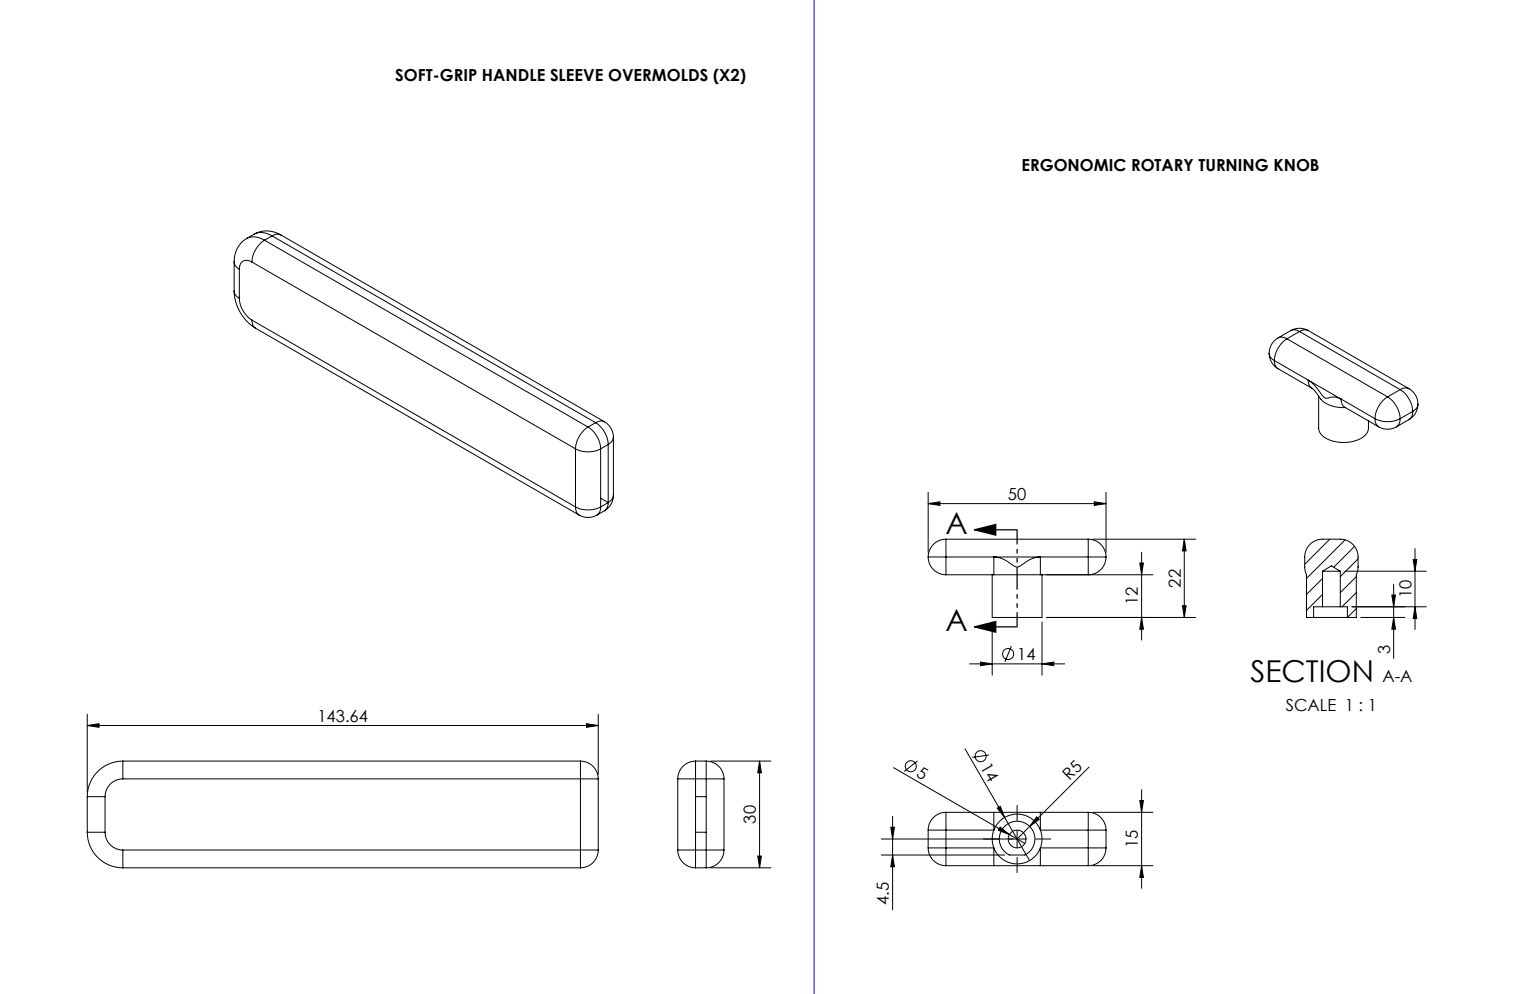
ISO-10303-21;
HEADER;
FILE_DESCRIPTION (('STEP AP214'),
    '1' );
FILE_NAME ('Soft-Grip Handle Sleeve Overmolds (x2).step',
    '2026-09-24T10:15:42',
    ( '' ),
    ( '' ),
    'SwSTEP 2.0',
    'SolidWorks 2026',
    '' );
FILE_SCHEMA (( 'AUTOMOTIVE_DESIGN' ));
ENDSEC;

DATA;
#10=DIRECTION ( 'NONE',  ( -0.000000000000000000, 1.000000000000000000, -0.000000000000000000 ) ) ;
#45=( NAMED_UNIT ( * ) PLANE_ANGLE_UNIT ( ) SI_UNIT ( $, .RADIAN. ) );
#53=DIRECTION ( 'NONE',  ( 0.000000000000000000, 0.000000000000000000, 1.000000000000000000 ) ) ;
#71=EDGE_CURVE ( 'NONE', #14216, #17792, #8218, .T. ) ;
#74=EDGE_CURVE ( 'NONE', #18124, #2507, #14609, .T. ) ;
#81=ORIENTED_EDGE ( 'NONE', *, *, #18589, .F. ) ;
#107=AXIS2_PLACEMENT_3D ( 'NONE', #8749, #9037, #10469 ) ;
#121=FACE_OUTER_BOUND ( 'NONE', #17396, .T. ) ;
#125=ORIENTED_EDGE ( 'NONE', *, *, #5943, .T. ) ;
#129=EDGE_CURVE ( 'NONE', #11279, #879, #18664, .T. ) ;
#146=( NAMED_UNIT ( * ) PLANE_ANGLE_UNIT ( ) SI_UNIT ( $, .RADIAN. ) );
#165=ORIENTED_EDGE ( 'NONE', *, *, #2738, .T. ) ;
#168=DIRECTION ( 'NONE',  ( 2.775557561562891351E-15, 0.000000000000000000, -1.000000000000000000 ) ) ;
#195=EDGE_CURVE ( 'NONE', #996, #10455, #10657, .T. ) ;
#204=VERTEX_POINT ( 'NONE', #4724 ) ;
#216=AXIS2_PLACEMENT_3D ( 'NONE', #4197, #14959, #10013 ) ;
#297=ADVANCED_FACE ( 'NONE', ( #11306 ), #18192, .T. ) ;
#339=( NAMED_UNIT ( * ) SI_UNIT ( $, .STERADIAN. ) SOLID_ANGLE_UNIT ( ) );
#364=CARTESIAN_POINT ( 'NONE',  ( -199.9999999999999716, -10.00000000000002665, 6.000000000000000000 ) ) ;
#368=PRODUCT_DEFINITION_SHAPE ( 'NONE', 'NONE',  #14430 ) ;
#400=VERTEX_POINT ( 'NONE', #4028 ) ;
#441=VECTOR ( 'NONE', #16423, 1000.000000000000000 ) ;
#456=ORIENTED_EDGE ( 'NONE', *, *, #3384, .T. ) ;
#478=DIRECTION ( 'NONE',  ( -1.000000000000000000, -1.298018465182616140E-16, -0.000000000000000000 ) ) ;
#495=ORIENTED_EDGE ( 'NONE', *, *, #13811, .F. ) ;
#571=ORIENTED_EDGE ( 'NONE', *, *, #13222, .F. ) ;
#632=DIRECTION ( 'NONE',  ( 0.000000000000000000, 0.000000000000000000, -1.000000000000000000 ) ) ;
#645=EDGE_CURVE ( 'NONE', #12951, #4745, #12694, .T. ) ;
#673=DIRECTION ( 'NONE',  ( 1.000000000000000000, 0.000000000000000000, -0.000000000000000000 ) ) ;
#681=AXIS2_PLACEMENT_3D ( 'NONE', #16263, #10, #9092 ) ;
#709=CYLINDRICAL_SURFACE ( 'NONE', #9338, 5.000000000000000000 ) ;
#710=CARTESIAN_POINT ( 'NONE',  ( -199.9999999999999716, -5.000000000000024869, 3.000000000000000000 ) ) ;
#723=EDGE_CURVE ( 'NONE', #14183, #11279, #13412, .T. ) ;
#729=EDGE_LOOP ( 'NONE', ( #5711, #14745, #14272, #12333 ) ) ;
#732=FACE_OUTER_BOUND ( 'NONE', #9253, .T. ) ;
#733=CARTESIAN_POINT ( 'NONE',  ( -66.35602477868049220, -15.00000000000001066, -153.7432847437423789 ) ) ;
#741=LINE ( 'NONE', #9527, #14448 ) ;
#746=ORIENTED_EDGE ( 'NONE', *, *, #8212, .T. ) ;
#763=LINE ( 'NONE', #18253, #3069 ) ;
#778=ORIENTED_EDGE ( 'NONE', *, *, #1912, .F. ) ;
#783=CARTESIAN_POINT ( 'NONE',  ( -194.9999999999999716, 4.999999999999973355, 6.000000000000000000 ) ) ;
#830=COLOUR_RGB ( '', 0.08235294, 0.09019608, 0.10196078) ;
#879=VERTEX_POINT ( 'NONE', #5706 ) ;
#880=DIRECTION ( 'NONE',  ( 1.000000000000000000, 1.298018465182616140E-16, 0.000000000000000000 ) ) ;
#921=LINE ( 'NONE', #8015, #14130 ) ;
#932=DIRECTION ( 'NONE',  ( -1.000000000000000000, 0.000000000000000000, 0.000000000000000000 ) ) ;
#947=ORIENTED_EDGE ( 'NONE', *, *, #11281, .T. ) ;
#949=EDGE_CURVE ( 'NONE', #14986, #8583, #5172, .T. ) ;
#979=LINE ( 'NONE', #3397, #6527 ) ;
#996=VERTEX_POINT ( 'NONE', #10503 ) ;
#1017=CARTESIAN_POINT ( 'NONE',  ( -194.9999999999999716, 4.999999999999973355, 11.00000000000000000 ) ) ;
#1053=CARTESIAN_POINT ( 'NONE',  ( -194.9999999999999716, -15.00000000000003020, -153.7432847437423789 ) ) ;
#1169=CARTESIAN_POINT ( 'NONE',  ( -194.9999999999999716, -10.00000000000002665, 11.00000000000000000 ) ) ;
#1263=CARTESIAN_POINT ( 'NONE',  ( -194.9999999999999716, 9.999999999999973355, 3.000000000000000000 ) ) ;
#1267=DIRECTION ( 'NONE',  ( -0.000000000000000000, -0.000000000000000000, 1.000000000000000000 ) ) ;
#1290=AXIS2_PLACEMENT_3D ( 'NONE', #1861, #1565, #7701 ) ;
#1301=CARTESIAN_POINT ( 'NONE',  ( -61.35602477868049220, 9.999999999999973355, 6.000000000000000000 ) ) ;
#1311=CARTESIAN_POINT ( 'NONE',  ( -61.35602477868047799, -10.00000000000000888, -153.7432847437423789 ) ) ;
#1312=EDGE_CURVE ( 'NONE', #1583, #8583, #4177, .T. ) ;
#1314=ORIENTED_EDGE ( 'NONE', *, *, #723, .T. ) ;
#1317=CYLINDRICAL_SURFACE ( 'NONE', #216, 5.000000000000000000 ) ;
#1334=CARTESIAN_POINT ( 'NONE',  ( 1.298018465182615993E-15, -10.00000000000000000, -2.000000000000000000 ) ) ;
#1355=CARTESIAN_POINT ( 'NONE',  ( 0.000000000000000000, 0.000000000000000000, 6.000000000000000000 ) ) ;
#1371=AXIS2_PLACEMENT_3D ( 'NONE', #17480, #5906, #4386 ) ;
#1389=DIRECTION ( 'NONE',  ( -0.000000000000000000, 0.000000000000000000, -1.000000000000000000 ) ) ;
#1393=ORIENTED_EDGE ( 'NONE', *, *, #11938, .T. ) ;
#1436=CARTESIAN_POINT ( 'NONE',  ( -194.9999999999999716, -10.00000000000002665, -2.000000000000000000 ) ) ;
#1460=CIRCLE ( 'NONE', #12158, 5.000000000000000000 ) ;
#1465=CARTESIAN_POINT ( 'NONE',  ( -66.35602477868047799, 9.999999999999973355, -2.000000000000000000 ) ) ;
#1474=EDGE_CURVE ( 'NONE', #11944, #7533, #979, .T. ) ;
#1485=CARTESIAN_POINT ( 'NONE',  ( -194.9999999999999716, 14.99999999999997513, 6.000000000000005329 ) ) ;
#1487=( LENGTH_UNIT ( ) NAMED_UNIT ( * ) SI_UNIT ( .MILLI., .METRE. ) );
#1496=ORIENTED_EDGE ( 'NONE', *, *, #18440, .T. ) ;
#1498=ORIENTED_EDGE ( 'NONE', *, *, #9213, .F. ) ;
#1512=DIRECTION ( 'NONE',  ( 0.000000000000000000, 0.000000000000000000, -1.000000000000000000 ) ) ;
#1558=ORIENTED_EDGE ( 'NONE', *, *, #2425, .T. ) ;
#1563=CARTESIAN_POINT ( 'NONE',  ( -194.9999999999999716, -10.00000000000002665, 6.000000000000000000 ) ) ;
#1565=DIRECTION ( 'NONE',  ( 0.000000000000000000, 0.000000000000000000, -1.000000000000000000 ) ) ;
#1583=VERTEX_POINT ( 'NONE', #11396 ) ;
#1593=CARTESIAN_POINT ( 'NONE',  ( -205.0000000000000000, 4.999999999999975131, 3.000000000000002665 ) ) ;
#1621=DIRECTION ( 'NONE',  ( 1.000000000000000000, 0.000000000000000000, 0.000000000000000000 ) ) ;
#1625=ORIENTED_EDGE ( 'NONE', *, *, #5264, .F. ) ;
#1702=ORIENTED_EDGE ( 'NONE', *, *, #5723, .T. ) ;
#1765=( LENGTH_UNIT ( ) NAMED_UNIT ( * ) SI_UNIT ( .MILLI., .METRE. ) );
#1782=ORIENTED_EDGE ( 'NONE', *, *, #7144, .F. ) ;
#1799=PLANE ( 'NONE',  #7889 ) ;
#1861=CARTESIAN_POINT ( 'NONE',  ( 0.000000000000000000, 0.000000000000000000, 3.000000000000000000 ) ) ;
#1912=EDGE_CURVE ( 'NONE', #15844, #11944, #5028, .T. ) ;
#2027=DIRECTION ( 'NONE',  ( -1.000000000000000000, 0.000000000000000000, 0.000000000000000000 ) ) ;
#2030=AXIS2_PLACEMENT_3D ( 'NONE', #15716, #11248, #17249 ) ;
#2035=DIRECTION ( 'NONE',  ( 1.000000000000000000, -0.000000000000000000, 0.000000000000000000 ) ) ;
#2097=EDGE_LOOP ( 'NONE', ( #13783, #6508, #11629, #2309 ) ) ;
#2114=DIRECTION ( 'NONE',  ( 0.000000000000000000, 0.000000000000000000, -1.000000000000000000 ) ) ;
#2149=CARTESIAN_POINT ( 'NONE',  ( -194.9999999999999716, -10.00000000000002665, 5.999999999999999112 ) ) ;
#2213=CYLINDRICAL_SURFACE ( 'NONE', #13097, 10.00000000000000888 ) ;
#2265=ORIENTED_EDGE ( 'NONE', *, *, #8107, .F. ) ;
#2286=LINE ( 'NONE', #16550, #9676 ) ;
#2293=CARTESIAN_POINT ( 'NONE',  ( -194.9999999999999716, -5.000000000000024869, 6.000000000000000000 ) ) ;
#2296=VERTEX_POINT ( 'NONE', #13247 ) ;
#2308=DIRECTION ( 'NONE',  ( -1.000000000000000000, 0.000000000000000000, 0.000000000000000000 ) ) ;
#2309=ORIENTED_EDGE ( 'NONE', *, *, #74, .F. ) ;
#2318=DIRECTION ( 'NONE',  ( -1.000000000000000000, 0.000000000000000000, 0.000000000000000000 ) ) ;
#2331=DIRECTION ( 'NONE',  ( 0.000000000000000000, 0.000000000000000000, 1.000000000000000000 ) ) ;
#2341=ORIENTED_EDGE ( 'NONE', *, *, #6570, .F. ) ;
#2349=CIRCLE ( 'NONE', #17297, 5.000000000000000000 ) ;
#2359=ORIENTED_EDGE ( 'NONE', *, *, #9146, .T. ) ;
#2365=CARTESIAN_POINT ( 'NONE',  ( -194.9999999999999716, -15.00000000000002665, -153.7432847437423789 ) ) ;
#2368=CARTESIAN_POINT ( 'NONE',  ( -194.9999999999999716, 9.999999999999976907, -2.000000000000000000 ) ) ;
#2401=ORIENTED_EDGE ( 'NONE', *, *, #9051, .T. ) ;
#2410=AXIS2_PLACEMENT_3D ( 'NONE', #3830, #2035, #12340 ) ;
#2417=CYLINDRICAL_SURFACE ( 'NONE', #2513, 4.999999999999997335 ) ;
#2425=EDGE_CURVE ( 'NONE', #4745, #12842, #13817, .T. ) ;
#2460=CIRCLE ( 'NONE', #3389, 5.000000000000004441 ) ;
#2462=ADVANCED_FACE ( 'NONE', ( #11521 ), #3966, .T. ) ;
#2496=UNCERTAINTY_MEASURE_WITH_UNIT (LENGTH_MEASURE( 1.000000000000000082E-05 ), #1765, 'distance_accuracy_value', 'NONE');
#2507=VERTEX_POINT ( 'NONE', #7414 ) ;
#2509=ORIENTED_EDGE ( 'NONE', *, *, #7144, .T. ) ;
#2513=AXIS2_PLACEMENT_3D ( 'NONE', #6741, #8534, #5291 ) ;
#2518=DIRECTION ( 'NONE',  ( 1.000000000000000000, 0.000000000000000000, 2.775557561562889773E-15 ) ) ;
#2538=AXIS2_PLACEMENT_3D ( 'NONE', #7054, #5593, #17264 ) ;
#2551=DIRECTION ( 'NONE',  ( 0.000000000000000000, 0.000000000000000000, -1.000000000000000000 ) ) ;
#2557=DIRECTION ( 'NONE',  ( 0.000000000000000000, 1.000000000000000000, 0.000000000000000000 ) ) ;
#2580=AXIS2_PLACEMENT_3D ( 'NONE', #13797, #8261, #5192 ) ;
#2594=DIRECTION ( 'NONE',  ( 1.000000000000000000, 0.000000000000000000, 0.000000000000000000 ) ) ;
#2641=LINE ( 'NONE', #18606, #10242 ) ;
#2659=ORIENTED_EDGE ( 'NONE', *, *, #17064, .F. ) ;
#2710=DIRECTION ( 'NONE',  ( 1.000000000000000000, 0.000000000000000000, 0.000000000000000000 ) ) ;
#2738=EDGE_CURVE ( 'NONE', #11944, #14183, #18292, .T. ) ;
#2752=CYLINDRICAL_SURFACE ( 'NONE', #18758, 5.000000000000000888 ) ;
#2780=CARTESIAN_POINT ( 'NONE',  ( -66.35602477868047799, -10.00000000000000888, -2.000000000000000000 ) ) ;
#2789=ORIENTED_EDGE ( 'NONE', *, *, #129, .T. ) ;
#2929=VECTOR ( 'NONE', #1389, 1000.000000000000000 ) ;
#2933=DIRECTION ( 'NONE',  ( 1.000000000000000000, -2.775557561562892929E-15, 0.000000000000000000 ) ) ;
#2954=ADVANCED_FACE ( 'NONE', ( #16249 ), #3131, .T. ) ;
#2956=ORIENTED_EDGE ( 'NONE', *, *, #18476, .F. ) ;
#2989=( NAMED_UNIT ( * ) SI_UNIT ( $, .STERADIAN. ) SOLID_ANGLE_UNIT ( ) );
#3005=EDGE_LOOP ( 'NONE', ( #15141, #81, #4937, #1625 ) ) ;
#3041=EDGE_LOOP ( 'NONE', ( #9922, #15624, #14342, #4151 ) ) ;
#3069=VECTOR ( 'NONE', #7854, 1000.000000000000000 ) ;
#3070=DIRECTION ( 'NONE',  ( 0.000000000000000000, 0.000000000000000000, -1.000000000000000000 ) ) ;
#3076=SURFACE_STYLE_USAGE ( .BOTH. , #10364 ) ;
#3084=LINE ( 'NONE', #10175, #6365 ) ;
#3124=SPHERICAL_SURFACE ( 'NONE', #14476, 5.000000000000000000 ) ;
#3131=SPHERICAL_SURFACE ( 'NONE', #5399, 5.000000000000000000 ) ;
#3159=EDGE_CURVE ( 'NONE', #4745, #5087, #16034, .T. ) ;
#3176=( NAMED_UNIT ( * ) SI_UNIT ( $, .STERADIAN. ) SOLID_ANGLE_UNIT ( ) );
#3183=DIRECTION ( 'NONE',  ( -0.000000000000000000, 1.000000000000000000, -0.000000000000000000 ) ) ;
#3198=CARTESIAN_POINT ( 'NONE',  ( -59.99999999999997158, -10.00000000000000888, 3.000000000000000000 ) ) ;
#3214=EDGE_LOOP ( 'NONE', ( #4994, #3976, #1782 ) ) ;
#3219=ORIENTED_EDGE ( 'NONE', *, *, #5723, .F. ) ;
#3234=DIRECTION ( 'NONE',  ( 0.000000000000000000, -1.000000000000000000, -0.000000000000000000 ) ) ;
#3259=MECHANICAL_DESIGN_GEOMETRIC_PRESENTATION_REPRESENTATION('',(#8169),#4186);
#3284=DIRECTION ( 'NONE',  ( -1.000000000000000000, -1.239088197126290570E-16, 0.000000000000000000 ) ) ;
#3306=CARTESIAN_POINT ( 'NONE',  ( -194.9999999999999716, -10.00000000000002665, 3.000000000000000000 ) ) ;
#3326=CIRCLE ( 'NONE', #2410, 5.000000000000000000 ) ;
#3355=CARTESIAN_POINT ( 'NONE',  ( -194.9999999999999716, 14.99999999999997513, -153.7432847437423789 ) ) ;
#3360=DIRECTION ( 'NONE',  ( 0.000000000000000000, 0.000000000000000000, 1.000000000000000000 ) ) ;
#3370=EDGE_LOOP ( 'NONE', ( #13830, #15289, #2956 ) ) ;
#3371=DIRECTION ( 'NONE',  ( 0.000000000000000000, 0.000000000000000000, 1.000000000000000000 ) ) ;
#3384=EDGE_CURVE ( 'NONE', #11365, #1583, #16163, .T. ) ;
#3386=APPLICATION_CONTEXT ( 'automotive_design' ) ;
#3389=AXIS2_PLACEMENT_3D ( 'NONE', #9370, #2114, #13759 ) ;
#3397=CARTESIAN_POINT ( 'NONE',  ( -199.9999999999999716, 4.999999999999973355, 6.000000000000000000 ) ) ;
#3488=VECTOR ( 'NONE', #1267, 1000.000000000000000 ) ;
#3542=VERTEX_POINT ( 'NONE', #710 ) ;
#3584=VECTOR ( 'NONE', #18387, 1000.000000000000000 ) ;
#3655=ORIENTED_EDGE ( 'NONE', *, *, #11968, .F. ) ;
#3672=DIRECTION ( 'NONE',  ( -1.239088197126290570E-16, 1.000000000000000000, 0.000000000000000000 ) ) ;
#3728=ORIENTED_EDGE ( 'NONE', *, *, #1474, .T. ) ;
#3773=AXIS2_PLACEMENT_3D ( 'NONE', #10326, #16152, #1621 ) ;
#3792=ORIENTED_EDGE ( 'NONE', *, *, #74, .T. ) ;
#3798=DIRECTION ( 'NONE',  ( 1.298018465182616140E-16, -1.000000000000000000, 0.000000000000000000 ) ) ;
#3808=CARTESIAN_POINT ( 'NONE',  ( -66.35602477868047799, 9.999999999999973355, 5.999999999999999112 ) ) ;
#3809=CARTESIAN_POINT ( 'NONE',  ( -205.0000000000000000, -5.000000000000024869, 6.000000000000005329 ) ) ;
#3829=VECTOR ( 'NONE', #11704, 1000.000000000000000 ) ;
#3830=CARTESIAN_POINT ( 'NONE',  ( -194.9999999999999716, 9.999999999999976907, 3.000000000000000000 ) ) ;
#3893=VERTEX_POINT ( 'NONE', #5074 ) ;
#3918=DIRECTION ( 'NONE',  ( -0.000000000000000000, -0.000000000000000000, 1.000000000000000000 ) ) ;
#3931=AXIS2_PLACEMENT_3D ( 'NONE', #4340, #14651, #14743 ) ;
#3940=ORIENTED_EDGE ( 'NONE', *, *, #13397, .F. ) ;
#3944=DIRECTION ( 'NONE',  ( 0.000000000000000000, 0.000000000000000000, -1.000000000000000000 ) ) ;
#3953=AXIS2_PLACEMENT_3D ( 'NONE', #5234, #15192, #932 ) ;
#3954=CARTESIAN_POINT ( 'NONE',  ( -199.9999999999999716, -5.000000000000024869, 3.000000000000000000 ) ) ;
#3966=CYLINDRICAL_SURFACE ( 'NONE', #7563, 4.999999999999997335 ) ;
#3976=ORIENTED_EDGE ( 'NONE', *, *, #3159, .T. ) ;
#4008=CARTESIAN_POINT ( 'NONE',  ( -199.9999999999999716, 4.999999999999974243, -2.000000000000000000 ) ) ;
#4028=CARTESIAN_POINT ( 'NONE',  ( -199.9999999999999716, 4.999999999999974243, 11.00000000000000000 ) ) ;
#4047=CARTESIAN_POINT ( 'NONE',  ( -194.9999999999999716, 9.999999999999973355, 6.000000000000000000 ) ) ;
#4062=CARTESIAN_POINT ( 'NONE',  ( -205.0000000000000000, 4.999999999999974243, 3.000000000000002665 ) ) ;
#4086=DIRECTION ( 'NONE',  ( -1.000000000000000000, 0.000000000000000000, 0.000000000000000000 ) ) ;
#4096=EDGE_CURVE ( 'NONE', #8123, #10867, #15534, .T. ) ;
#4114=CARTESIAN_POINT ( 'NONE',  ( -194.9999999999999716, 9.999999999999973355, 3.000000000000002665 ) ) ;
#4151=ORIENTED_EDGE ( 'NONE', *, *, #11967, .T. ) ;
#4156=EDGE_LOOP ( 'NONE', ( #15184, #15990, #2659, #571 ) ) ;
#4157=AXIS2_PLACEMENT_3D ( 'NONE', #1017, #8029, #8208 ) ;
#4177=LINE ( 'NONE', #13436, #12921 ) ;
#4179=DIRECTION ( 'NONE',  ( 1.000000000000000000, 0.000000000000000000, -0.000000000000000000 ) ) ;
#4186=( GEOMETRIC_REPRESENTATION_CONTEXT ( 3 ) GLOBAL_UNCERTAINTY_ASSIGNED_CONTEXT ( ( #2496 ) ) GLOBAL_UNIT_ASSIGNED_CONTEXT ( ( #1765, #6067, #3176 ) ) REPRESENTATION_CONTEXT ( 'NONE', 'WORKASPACE' ) );
#4189=CLOSED_SHELL ( 'NONE', ( #297, #7987, #9459, #11355, #4727, #17066, #8467, #18898, #9820, #4892, #7667, #11879, #11295, #14268, #8812, #8260, #18591, #14598, #18465, #18406, #2462, #16106, #2954, #16000, #18217, #9314, #7143, #4861, #13549, #11149, #9662, #7236 ) ) ;
#4197=CARTESIAN_POINT ( 'NONE',  ( -199.9999999999999716, 4.999999999999975131, 3.000000000000002665 ) ) ;
#4238=EDGE_CURVE ( 'NONE', #14839, #12842, #11714, .T. ) ;
#4260=DIRECTION ( 'NONE',  ( 0.000000000000000000, 0.000000000000000000, 1.000000000000000000 ) ) ;
#4297=CYLINDRICAL_SURFACE ( 'NONE', #1371, 5.000000000000000000 ) ;
#4298=VERTEX_POINT ( 'NONE', #2368 ) ;
#4340=CARTESIAN_POINT ( 'NONE',  ( -194.9999999999999716, 4.999999999999973355, 3.000000000000002665 ) ) ;
#4375=SPHERICAL_SURFACE ( 'NONE', #8750, 5.000000000000000000 ) ;
#4381=VECTOR ( 'NONE', #10253, 1000.000000000000000 ) ;
#4386=DIRECTION ( 'NONE',  ( 0.000000000000000000, 1.000000000000000000, 0.000000000000000000 ) ) ;
#4388=DIRECTION ( 'NONE',  ( 1.000000000000000000, 0.000000000000000000, 0.000000000000000000 ) ) ;
#4423=ORIENTED_EDGE ( 'NONE', *, *, #10269, .T. ) ;
#4432=CARTESIAN_POINT ( 'NONE',  ( -194.9999999999999716, -5.000000000000024869, 6.000000000000000000 ) ) ;
#4443=AXIS2_PLACEMENT_3D ( 'NONE', #11088, #12592, #9464 ) ;
#4458=AXIS2_PLACEMENT_3D ( 'NONE', #7767, #17893, #2027 ) ;
#4487=ORIENTED_EDGE ( 'NONE', *, *, #14077, .T. ) ;
#4501=VECTOR ( 'NONE', #880, 1000.000000000000000 ) ;
#4539=EDGE_CURVE ( 'NONE', #10086, #3893, #6235, .T. ) ;
#4553=ORIENTED_EDGE ( 'NONE', *, *, #9404, .T. ) ;
#4573=FACE_OUTER_BOUND ( 'NONE', #3370, .T. ) ;
#4585=DIRECTION ( 'NONE',  ( 0.000000000000000000, 0.000000000000000000, -1.000000000000000000 ) ) ;
#4614=EDGE_CURVE ( 'NONE', #17792, #996, #7535, .T. ) ;
#4670=EDGE_CURVE ( 'NONE', #18124, #4997, #12934, .T. ) ;
#4671=ORIENTED_EDGE ( 'NONE', *, *, #1912, .T. ) ;
#4682=CIRCLE ( 'NONE', #15046, 5.000000000000000000 ) ;
#4685=DIRECTION ( 'NONE',  ( 0.000000000000000000, 0.000000000000000000, -1.000000000000000000 ) ) ;
#4686=CARTESIAN_POINT ( 'NONE',  ( -194.9999999999999716, -15.00000000000003020, 6.000000000000005329 ) ) ;
#4688=EDGE_CURVE ( 'NONE', #2296, #14986, #4708, .T. ) ;
#4700=ORIENTED_EDGE ( 'NONE', *, *, #12074, .F. ) ;
#4708=CIRCLE ( 'NONE', #15382, 5.000000000000000000 ) ;
#4724=CARTESIAN_POINT ( 'NONE',  ( -66.35602477868049220, -10.00000000000000888, 11.00000000000000000 ) ) ;
#4725=EDGE_LOOP ( 'NONE', ( #2509, #11743, #18683, #495 ) ) ;
#4727=ADVANCED_FACE ( 'NONE', ( #4944 ), #6474, .T. ) ;
#4729=FILL_AREA_STYLE ('',( #17632 ) ) ;
#4745=VERTEX_POINT ( 'NONE', #15658 ) ;
#4747=VERTEX_POINT ( 'NONE', #4008 ) ;
#4749=VECTOR ( 'NONE', #18648, 1000.000000000000000 ) ;
#4762=CARTESIAN_POINT ( 'NONE',  ( -66.35602477868047799, 9.999999999999973355, 5.999999999999999112 ) ) ;
#4763=ORIENTED_EDGE ( 'NONE', *, *, #12688, .T. ) ;
#4777=AXIS2_PLACEMENT_3D ( 'NONE', #6838, #8006, #15436 ) ;
#4812=LINE ( 'NONE', #15468, #10950 ) ;
#4835=LINE ( 'NONE', #1334, #16033 ) ;
#4844=ORIENTED_EDGE ( 'NONE', *, *, #4688, .F. ) ;
#4861=ADVANCED_FACE ( 'NONE', ( #13174 ), #5904, .T. ) ;
#4865=ORIENTED_EDGE ( 'NONE', *, *, #11732, .F. ) ;
#4892=ADVANCED_FACE ( 'NONE', ( #13268 ), #8875, .T. ) ;
#4897=ORIENTED_EDGE ( 'NONE', *, *, #15609, .F. ) ;
#4937=ORIENTED_EDGE ( 'NONE', *, *, #17064, .T. ) ;
#4944=FACE_OUTER_BOUND ( 'NONE', #14107, .T. ) ;
#4970=FACE_OUTER_BOUND ( 'NONE', #2097, .T. ) ;
#4982=EDGE_LOOP ( 'NONE', ( #16888, #8730, #17424, #4423, #3792, #15660 ) ) ;
#4994=ORIENTED_EDGE ( 'NONE', *, *, #645, .T. ) ;
#4997=VERTEX_POINT ( 'NONE', #15605 ) ;
#5028=CIRCLE ( 'NONE', #17535, 5.000000000000004441 ) ;
#5035=CARTESIAN_POINT ( 'NONE',  ( -199.9999999999999716, -10.00000000000002665, 3.000000000000000000 ) ) ;
#5048=FACE_OUTER_BOUND ( 'NONE', #12747, .T. ) ;
#5050=EDGE_CURVE ( 'NONE', #11395, #15844, #11233, .T. ) ;
#5074=CARTESIAN_POINT ( 'NONE',  ( -194.9999999999999716, 9.999999999999973355, 11.00000000000000000 ) ) ;
#5087=VERTEX_POINT ( 'NONE', #2780 ) ;
#5109=PRODUCT_CONTEXT ( 'NONE', #8042, 'mechanical' ) ;
#5172=CIRCLE ( 'NONE', #5770, 5.000000000000000000 ) ;
#5177=CARTESIAN_POINT ( 'NONE',  ( -194.9999999999999716, 14.99999999999997513, 3.000000000000002665 ) ) ;
#5179=CARTESIAN_POINT ( 'NONE',  ( -194.9999999999999716, -15.00000000000002665, 3.000000000000002665 ) ) ;
#5192=DIRECTION ( 'NONE',  ( 0.000000000000000000, 0.000000000000000000, 1.000000000000000000 ) ) ;
#5224=CARTESIAN_POINT ( 'NONE',  ( -199.9999999999999716, 4.999999999999973355, 6.000000000000000000 ) ) ;
#5234=CARTESIAN_POINT ( 'NONE',  ( -66.35602477868047799, 9.999999999999973355, 3.000000000000002665 ) ) ;
#5235=DIRECTION ( 'NONE',  ( 1.000000000000000000, 1.298018465182616140E-16, 0.000000000000000000 ) ) ;
#5264=EDGE_CURVE ( 'NONE', #11365, #14216, #12347, .T. ) ;
#5285=AXIS2_PLACEMENT_3D ( 'NONE', #8439, #2331, #2594 ) ;
#5291=DIRECTION ( 'NONE',  ( 1.000000000000000000, 0.000000000000000000, 0.000000000000000000 ) ) ;
#5297=ORIENTED_EDGE ( 'NONE', *, *, #13444, .F. ) ;
#5307=AXIS2_PLACEMENT_3D ( 'NONE', #3306, #9148, #10388 ) ;
#5334=CARTESIAN_POINT ( 'NONE',  ( -66.35602477868047799, -15.00000000000001066, 3.000000000000002665 ) ) ;
#5358=TOROIDAL_SURFACE ( 'NONE', #12676, 5.000000000000005329, 5.000000000000000000 ) ;
#5384=DIRECTION ( 'NONE',  ( 0.000000000000000000, 1.000000000000000000, 0.000000000000000000 ) ) ;
#5390=CIRCLE ( 'NONE', #7858, 5.000000000000000888 ) ;
#5399=AXIS2_PLACEMENT_3D ( 'NONE', #6409, #7851, #4685 ) ;
#5409=CARTESIAN_POINT ( 'NONE',  ( -61.35602477868047799, -10.00000000000000888, 6.000000000000000000 ) ) ;
#5466=EDGE_LOOP ( 'NONE', ( #2341, #1496, #6560 ) ) ;
#5482=CARTESIAN_POINT ( 'NONE',  ( -66.35602477868047799, 9.999999999999973355, 3.000000000000002665 ) ) ;
#5523=CARTESIAN_POINT ( 'NONE',  ( -66.35602477868049220, 9.999999999999973355, 5.999999999999999112 ) ) ;
#5558=ORIENTED_EDGE ( 'NONE', *, *, #9939, .F. ) ;
#5575=DIRECTION ( 'NONE',  ( 1.000000000000000000, 0.000000000000000000, 0.000000000000000000 ) ) ;
#5580=VECTOR ( 'NONE', #10132, 1000.000000000000000 ) ;
#5593=DIRECTION ( 'NONE',  ( 1.000000000000000000, 0.000000000000000000, 0.000000000000000000 ) ) ;
#5610=EDGE_CURVE ( 'NONE', #1583, #11395, #2286, .T. ) ;
#5643=DIRECTION ( 'NONE',  ( -0.000000000000000000, -1.000000000000000000, -0.000000000000000000 ) ) ;
#5669=CARTESIAN_POINT ( 'NONE',  ( -61.35602477868047799, -15.00000000000001066, 3.000000000000002665 ) ) ;
#5706=CARTESIAN_POINT ( 'NONE',  ( -194.9999999999999716, -10.00000000000002665, 3.000000000000000000 ) ) ;
#5711=ORIENTED_EDGE ( 'NONE', *, *, #14301, .F. ) ;
#5723=EDGE_CURVE ( 'NONE', #10455, #8123, #5390, .T. ) ;
#5742=DIRECTION ( 'NONE',  ( 0.000000000000000000, 1.000000000000000000, 0.000000000000000000 ) ) ;
#5770=AXIS2_PLACEMENT_3D ( 'NONE', #5523, #14329, #18710 ) ;
#5791=SPHERICAL_SURFACE ( 'NONE', #12083, 5.000000000000000000 ) ;
#5865=SURFACE_STYLE_FILL_AREA ( #7616 ) ;
#5904=PLANE ( 'NONE',  #9883 ) ;
#5906=DIRECTION ( 'NONE',  ( 1.000000000000000000, 1.298018465182616140E-16, 0.000000000000000000 ) ) ;
#5929=UNCERTAINTY_MEASURE_WITH_UNIT (LENGTH_MEASURE( 1.000000000000000082E-05 ), #1487, 'distance_accuracy_value', 'NONE');
#5943=EDGE_CURVE ( 'NONE', #10455, #14367, #15247, .T. ) ;
#5968=PRESENTATION_STYLE_ASSIGNMENT (( #16302 ) ) ;
#5983=( GEOMETRIC_REPRESENTATION_CONTEXT ( 3 ) GLOBAL_UNCERTAINTY_ASSIGNED_CONTEXT ( ( #8993 ) ) GLOBAL_UNIT_ASSIGNED_CONTEXT ( ( #16404, #146, #2989 ) ) REPRESENTATION_CONTEXT ( 'NONE', 'WORKASPACE' ) );
#6003=ORIENTED_EDGE ( 'NONE', *, *, #3159, .F. ) ;
#6017=ORIENTED_EDGE ( 'NONE', *, *, #949, .F. ) ;
#6063=DIRECTION ( 'NONE',  ( 0.000000000000000000, 0.000000000000000000, -1.000000000000000000 ) ) ;
#6067=( NAMED_UNIT ( * ) PLANE_ANGLE_UNIT ( ) SI_UNIT ( $, .RADIAN. ) );
#6102=FACE_OUTER_BOUND ( 'NONE', #8541, .T. ) ;
#6161=ORIENTED_EDGE ( 'NONE', *, *, #13811, .T. ) ;
#6191=DIRECTION ( 'NONE',  ( 1.000000000000000000, 0.000000000000000000, 0.000000000000000000 ) ) ;
#6235=CIRCLE ( 'NONE', #2538, 5.000000000000000000 ) ;
#6305=CARTESIAN_POINT ( 'NONE',  ( -199.9999999999999716, 4.999999999999973355, 5.999999999999999112 ) ) ;
#6355=ORIENTED_EDGE ( 'NONE', *, *, #195, .T. ) ;
#6357=ORIENTED_EDGE ( 'NONE', *, *, #13275, .T. ) ;
#6365=VECTOR ( 'NONE', #3183, 1000.000000000000000 ) ;
#6409=CARTESIAN_POINT ( 'NONE',  ( -66.35602477868047799, 9.999999999999973355, 3.000000000000000000 ) ) ;
#6429=DIRECTION ( 'NONE',  ( 1.000000000000000000, 0.000000000000000000, 0.000000000000000000 ) ) ;
#6460=VECTOR ( 'NONE', #14318, 1000.000000000000000 ) ;
#6474=PLANE ( 'NONE',  #17836 ) ;
#6508=ORIENTED_EDGE ( 'NONE', *, *, #13275, .F. ) ;
#6527=VECTOR ( 'NONE', #3944, 1000.000000000000000 ) ;
#6537=ORIENTED_EDGE ( 'NONE', *, *, #7881, .F. ) ;
#6560=ORIENTED_EDGE ( 'NONE', *, *, #4238, .F. ) ;
#6564=CYLINDRICAL_SURFACE ( 'NONE', #4777, 5.000000000000000000 ) ;
#6565=DIRECTION ( 'NONE',  ( -0.000000000000000000, 0.000000000000000000, 1.000000000000000000 ) ) ;
#6567=CARTESIAN_POINT ( 'NONE',  ( -59.99999999999997158, -10.00000000000000888, 6.000000000000000000 ) ) ;
#6569=VECTOR ( 'NONE', #478, 1000.000000000000000 ) ;
#6570=EDGE_CURVE ( 'NONE', #204, #14839, #14091, .T. ) ;
#6573=CARTESIAN_POINT ( 'NONE',  ( -194.9999999999999716, -10.00000000000003020, 11.00000000000000000 ) ) ;
#6576=DIRECTION ( 'NONE',  ( 0.000000000000000000, 0.000000000000000000, 1.000000000000000000 ) ) ;
#6582=AXIS2_PLACEMENT_3D ( 'NONE', #3355, #13300, #13203 ) ;
#6616=DIRECTION ( 'NONE',  ( 0.000000000000000000, 0.000000000000000000, -1.000000000000000000 ) ) ;
#6658=ORIENTED_EDGE ( 'NONE', *, *, #1474, .F. ) ;
#6684=PLANE ( 'NONE',  #13921 ) ;
#6741=CARTESIAN_POINT ( 'NONE',  ( -66.35602477868049220, -10.00000000000000888, -153.7432847437423789 ) ) ;
#6748=CARTESIAN_POINT ( 'NONE',  ( -205.0000000000000000, 4.999999999999975131, 6.000000000000005329 ) ) ;
#6751=ORIENTED_EDGE ( 'NONE', *, *, #6570, .T. ) ;
#6805=ORIENTED_EDGE ( 'NONE', *, *, #13397, .T. ) ;
#6838=CARTESIAN_POINT ( 'NONE',  ( -194.9999999999999716, 9.999999999999973355, 5.999999999999999112 ) ) ;
#6876=VECTOR ( 'NONE', #12112, 1000.000000000000000 ) ;
#6895=DIRECTION ( 'NONE',  ( 0.000000000000000000, 0.000000000000000000, 1.000000000000000000 ) ) ;
#6901=DIRECTION ( 'NONE',  ( -1.000000000000000000, 0.000000000000000000, -0.000000000000000000 ) ) ;
#6945=CARTESIAN_POINT ( 'NONE',  ( -199.9999999999999716, -5.000000000000024869, 6.000000000000000000 ) ) ;
#6947=CARTESIAN_POINT ( 'NONE',  ( -194.9999999999999716, -5.000000000000024869, 6.000000000000005329 ) ) ;
#6975=ORIENTED_EDGE ( 'NONE', *, *, #10269, .F. ) ;
#6989=DIRECTION ( 'NONE',  ( 0.000000000000000000, 0.000000000000000000, 1.000000000000000000 ) ) ;
#7033=DIRECTION ( 'NONE',  ( 2.775557561562891351E-15, 0.000000000000000000, -1.000000000000000000 ) ) ;
#7054=CARTESIAN_POINT ( 'NONE',  ( -194.9999999999999716, 9.999999999999976907, 6.000000000000005329 ) ) ;
#7126=FACE_OUTER_BOUND ( 'NONE', #18557, .T. ) ;
#7143=ADVANCED_FACE ( 'NONE', ( #16189 ), #13414, .F. ) ;
#7144=EDGE_CURVE ( 'NONE', #12951, #5087, #10766, .T. ) ;
#7179=AXIS2_PLACEMENT_3D ( 'NONE', #783, #6616, #18086 ) ;
#7198=DIRECTION ( 'NONE',  ( 0.000000000000000000, 0.000000000000000000, -1.000000000000000000 ) ) ;
#7207=( GEOMETRIC_REPRESENTATION_CONTEXT ( 3 ) GLOBAL_UNCERTAINTY_ASSIGNED_CONTEXT ( ( #5929 ) ) GLOBAL_UNIT_ASSIGNED_CONTEXT ( ( #1487, #45, #339 ) ) REPRESENTATION_CONTEXT ( 'NONE', 'WORKASPACE' ) );
#7215=ORIENTED_EDGE ( 'NONE', *, *, #2738, .F. ) ;
#7221=EDGE_LOOP ( 'NONE', ( #4487, #6537, #18328, #12753 ) ) ;
#7236=ADVANCED_FACE ( 'NONE', ( #11695 ), #17523, .F. ) ;
#7270=DIRECTION ( 'NONE',  ( -0.000000000000000000, -0.000000000000000000, 1.000000000000000000 ) ) ;
#7336=ORIENTED_EDGE ( 'NONE', *, *, #5050, .F. ) ;
#7409=ORIENTED_EDGE ( 'NONE', *, *, #5610, .T. ) ;
#7414=CARTESIAN_POINT ( 'NONE',  ( -199.9999999999999716, -5.000000000000024869, -2.000000000000000000 ) ) ;
#7416=CARTESIAN_POINT ( 'NONE',  ( -199.9999999999999716, 4.999999999999973355, 11.00000000000000000 ) ) ;
#7427=AXIS2_PLACEMENT_3D ( 'NONE', #11524, #12849, #2710 ) ;
#7430=ORIENTED_EDGE ( 'NONE', *, *, #4096, .T. ) ;
#7436=DIRECTION ( 'NONE',  ( 1.000000000000000000, -0.000000000000000000, 2.775557561562891351E-15 ) ) ;
#7441=TOROIDAL_SURFACE ( 'NONE', #3773, 5.000000000000005329, 5.000000000000000000 ) ;
#7517=CARTESIAN_POINT ( 'NONE',  ( -59.99999999999997158, -10.00000000000000888, 6.000000000000000000 ) ) ;
#7520=CARTESIAN_POINT ( 'NONE',  ( -66.35602477868049220, 9.999999999999973355, 11.00000000000000000 ) ) ;
#7533=VERTEX_POINT ( 'NONE', #18620 ) ;
#7535=LINE ( 'NONE', #1593, #441 ) ;
#7553=AXIS2_PLACEMENT_3D ( 'NONE', #13949, #2551, #8401 ) ;
#7561=ORIENTED_EDGE ( 'NONE', *, *, #11967, .F. ) ;
#7563=AXIS2_PLACEMENT_3D ( 'NONE', #17340, #18488, #8640 ) ;
#7607=CARTESIAN_POINT ( 'NONE',  ( -66.35602477868047799, -10.00000000000000888, 3.000000000000000000 ) ) ;
#7616=FILL_AREA_STYLE ('',( #13327 ) ) ;
#7635=AXIS2_PLACEMENT_3D ( 'NONE', #2293, #3918, #12702 ) ;
#7637=CARTESIAN_POINT ( 'NONE',  ( -61.35602477868047799, -10.00000000000000888, 3.000000000000000000 ) ) ;
#7667=ADVANCED_FACE ( 'NONE', ( #16343 ), #3124, .T. ) ;
#7695=CARTESIAN_POINT ( 'NONE',  ( -66.35602477868047799, 9.999999999999973355, 3.000000000000000000 ) ) ;
#7701=DIRECTION ( 'NONE',  ( -1.000000000000000000, 0.000000000000000000, -0.000000000000000000 ) ) ;
#7708=PRODUCT ( 'Soft-Grip Handle Sleeve Overmolds (x2)', 'Soft-Grip Handle Sleeve Overmolds (x2)', '', ( #5109 ) ) ;
#7740=ORIENTED_EDGE ( 'NONE', *, *, #1312, .T. ) ;
#7767=CARTESIAN_POINT ( 'NONE',  ( -66.35602477868047799, -10.00000000000000888, 3.000000000000002665 ) ) ;
#7818=EDGE_LOOP ( 'NONE', ( #11740, #16870, #16374, #3940 ) ) ;
#7823=AXIS2_PLACEMENT_3D ( 'NONE', #11155, #2518, #7033 ) ;
#7828=DIRECTION ( 'NONE',  ( 1.000000000000000000, 1.239088197126290570E-16, -0.000000000000000000 ) ) ;
#7843=CARTESIAN_POINT ( 'NONE',  ( -194.9999999999999716, -15.00000000000002665, 6.000000000000005329 ) ) ;
#7848=DIRECTION ( 'NONE',  ( 0.000000000000000000, -0.000000000000000000, -1.000000000000000000 ) ) ;
#7851=DIRECTION ( 'NONE',  ( -0.000000000000000000, 1.000000000000000000, 0.000000000000000000 ) ) ;
#7854=DIRECTION ( 'NONE',  ( -0.000000000000000000, -1.000000000000000000, -0.000000000000000000 ) ) ;
#7858=AXIS2_PLACEMENT_3D ( 'NONE', #18611, #9642, #53 ) ;
#7881=EDGE_CURVE ( 'NONE', #12842, #18304, #8025, .T. ) ;
#7889=AXIS2_PLACEMENT_3D ( 'NONE', #364, #6191, #16430 ) ;
#7908=CARTESIAN_POINT ( 'NONE',  ( -194.9999999999999716, -10.00000000000003020, 5.999999999999999112 ) ) ;
#7987=ADVANCED_FACE ( 'NONE', ( #12581 ), #18410, .T. ) ;
#8006=DIRECTION ( 'NONE',  ( -1.000000000000000000, 0.000000000000000000, 0.000000000000000000 ) ) ;
#8015=CARTESIAN_POINT ( 'NONE',  ( -61.35602477868047799, -15.00000000000001066, 6.000000000000005329 ) ) ;
#8025=LINE ( 'NONE', #7843, #6569 ) ;
#8029=DIRECTION ( 'NONE',  ( 0.000000000000000000, 0.000000000000000000, 1.000000000000000000 ) ) ;
#8037=DIRECTION ( 'NONE',  ( -0.000000000000000000, -0.000000000000000000, -1.000000000000000000 ) ) ;
#8039=CARTESIAN_POINT ( 'NONE',  ( -194.9999999999999716, -5.000000000000024869, 3.000000000000002665 ) ) ;
#8042=APPLICATION_CONTEXT ( 'automotive_design' ) ;
#8075=AXIS2_PLACEMENT_3D ( 'NONE', #14705, #6989, #4388 ) ;
#8107=EDGE_CURVE ( 'NONE', #879, #12951, #10480, .T. ) ;
#8117=AXIS2_PLACEMENT_3D ( 'NONE', #13758, #673, #12241 ) ;
#8123=VERTEX_POINT ( 'NONE', #15064 ) ;
#8135=FACE_OUTER_BOUND ( 'NONE', #4156, .T. ) ;
#8169=STYLED_ITEM ( 'NONE', ( #16396 ), #16668 ) ;
#8185=ORIENTED_EDGE ( 'NONE', *, *, #10971, .F. ) ;
#8208=DIRECTION ( 'NONE',  ( 1.000000000000000000, 0.000000000000000000, 0.000000000000000000 ) ) ;
#8212=EDGE_CURVE ( 'NONE', #14986, #3893, #8504, .T. ) ;
#8218=CIRCLE ( 'NONE', #3931, 10.00000000000000888 ) ;
#8223=CARTESIAN_POINT ( 'NONE',  ( -205.0000000000000000, 4.999999999999974243, 6.000000000000005329 ) ) ;
#8234=EDGE_LOOP ( 'NONE', ( #1314, #2789, #15805, #17945 ) ) ;
#8260=ADVANCED_FACE ( 'NONE', ( #17383 ), #4297, .T. ) ;
#8261=DIRECTION ( 'NONE',  ( 0.000000000000000000, 1.000000000000000000, 0.000000000000000000 ) ) ;
#8363=AXIS2_PLACEMENT_3D ( 'NONE', #14904, #7848, #10802 ) ;
#8401=DIRECTION ( 'NONE',  ( -1.000000000000000000, 0.000000000000000000, 0.000000000000000000 ) ) ;
#8435=EDGE_CURVE ( 'NONE', #3893, #400, #11181, .T. ) ;
#8439=CARTESIAN_POINT ( 'NONE',  ( -194.9999999999999716, 4.999999999999973355, -153.7432847437423789 ) ) ;
#8450=TOROIDAL_SURFACE ( 'NONE', #7553, 5.000000000000005329, 5.000000000000000000 ) ;
#8458=DIRECTION ( 'NONE',  ( 0.000000000000000000, 0.000000000000000000, 1.000000000000000000 ) ) ;
#8467=ADVANCED_FACE ( 'NONE', ( #5048 ), #6684, .T. ) ;
#8504=LINE ( 'NONE', #13080, #15123 ) ;
#8511=DIRECTION ( 'NONE',  ( -1.000000000000000000, 0.000000000000000000, 0.000000000000000000 ) ) ;
#8534=DIRECTION ( 'NONE',  ( -0.000000000000000000, 0.000000000000000000, 1.000000000000000000 ) ) ;
#8541=EDGE_LOOP ( 'NONE', ( #165, #5558, #11197, #6658 ) ) ;
#8576=DIRECTION ( 'NONE',  ( 1.444447458290427415E-30, 5.204170427930420297E-16, 1.000000000000000000 ) ) ;
#8583=VERTEX_POINT ( 'NONE', #1301 ) ;
#8594=ORIENTED_EDGE ( 'NONE', *, *, #13444, .T. ) ;
#8640=DIRECTION ( 'NONE',  ( 1.000000000000000000, 0.000000000000000000, 0.000000000000000000 ) ) ;
#8685=DIRECTION ( 'NONE',  ( 0.000000000000000000, 0.000000000000000000, 1.000000000000000000 ) ) ;
#8686=DIRECTION ( 'NONE',  ( -1.000000000000000000, 0.000000000000000000, 0.000000000000000000 ) ) ;
#8718=ORIENTED_EDGE ( 'NONE', *, *, #8435, .T. ) ;
#8723=LINE ( 'NONE', #8817, #4381 ) ;
#8730=ORIENTED_EDGE ( 'NONE', *, *, #18589, .T. ) ;
#8749=CARTESIAN_POINT ( 'NONE',  ( -194.9999999999999716, 4.999999999999973355, 6.000000000000005329 ) ) ;
#8750=AXIS2_PLACEMENT_3D ( 'NONE', #4762, #17861, #14982 ) ;
#8786=DIRECTION ( 'NONE',  ( 0.000000000000000000, 0.000000000000000000, 1.000000000000000000 ) ) ;
#8812=ADVANCED_FACE ( 'NONE', ( #732 ), #6564, .T. ) ;
#8817=CARTESIAN_POINT ( 'NONE',  ( -205.0000000000000000, 4.999999999999974243, -153.7432847437423789 ) ) ;
#8875=CYLINDRICAL_SURFACE ( 'NONE', #17217, 5.000000000000000000 ) ;
#8929=FACE_OUTER_BOUND ( 'NONE', #17525, .T. ) ;
#8993=UNCERTAINTY_MEASURE_WITH_UNIT (LENGTH_MEASURE( 1.000000000000000082E-05 ), #16404, 'distance_accuracy_value', 'NONE');
#9037=DIRECTION ( 'NONE',  ( -0.000000000000000000, -0.000000000000000000, -1.000000000000000000 ) ) ;
#9051=EDGE_CURVE ( 'NONE', #1583, #15356, #9945, .T. ) ;
#9092=DIRECTION ( 'NONE',  ( 0.000000000000000000, 0.000000000000000000, -1.000000000000000000 ) ) ;
#9125=LINE ( 'NONE', #10267, #14531 ) ;
#9146=EDGE_CURVE ( 'NONE', #204, #14986, #9125, .T. ) ;
#9148=DIRECTION ( 'NONE',  ( -1.000000000000000000, -0.000000000000000000, -0.000000000000000000 ) ) ;
#9196=CIRCLE ( 'NONE', #14989, 10.00000000000000888 ) ;
#9213=EDGE_CURVE ( 'NONE', #4747, #17792, #13585, .T. ) ;
#9242=PRODUCT_DEFINITION_CONTEXT ( 'detailed design', #3386, 'design' ) ;
#9253=EDGE_LOOP ( 'NONE', ( #10673, #14817, #4844, #7561 ) ) ;
#9314=ADVANCED_FACE ( 'NONE', ( #12276 ), #14446, .T. ) ;
#9338=AXIS2_PLACEMENT_3D ( 'NONE', #2149, #15142, #2557 ) ;
#9351=STYLED_ITEM ( 'NONE', ( #5968 ), #17679 ) ;
#9370=CARTESIAN_POINT ( 'NONE',  ( -194.9999999999999716, 4.999999999999973355, -2.000000000000000000 ) ) ;
#9404=EDGE_CURVE ( 'NONE', #10867, #204, #14270, .T. ) ;
#9419=AXIS2_PLACEMENT_3D ( 'NONE', #15502, #13880, #12357 ) ;
#9459=ADVANCED_FACE ( 'NONE', ( #14639 ), #14727, .T. ) ;
#9464=DIRECTION ( 'NONE',  ( -1.000000000000000000, 0.000000000000000000, 0.000000000000000000 ) ) ;
#9496=ORIENTED_EDGE ( 'NONE', *, *, #4539, .F. ) ;
#9527=CARTESIAN_POINT ( 'NONE',  ( -194.9999999999999716, 14.99999999999997513, 6.000000000000005329 ) ) ;
#9639=MECHANICAL_DESIGN_GEOMETRIC_PRESENTATION_REPRESENTATION('',(#9351),#7207);
#9642=DIRECTION ( 'NONE',  ( 0.000000000000000000, 1.000000000000000000, -0.000000000000000000 ) ) ;
#9657=DIRECTION ( 'NONE',  ( 0.000000000000000000, 0.000000000000000000, 1.000000000000000000 ) ) ;
#9662=ADVANCED_FACE ( 'NONE', ( #13864 ), #11014, .F. ) ;
#9672=DIRECTION ( 'NONE',  ( 0.000000000000000000, -1.040834085586084257E-15, -1.000000000000000000 ) ) ;
#9676=VECTOR ( 'NONE', #12245, 1000.000000000000000 ) ;
#9811=LINE ( 'NONE', #1311, #6460 ) ;
#9820=ADVANCED_FACE ( 'NONE', ( #10848 ), #709, .T. ) ;
#9825=DIRECTION ( 'NONE',  ( 0.000000000000000000, -0.000000000000000000, -1.000000000000000000 ) ) ;
#9867=ORIENTED_EDGE ( 'NONE', *, *, #8107, .T. ) ;
#9874=PRODUCT_DEFINITION_FORMATION_WITH_SPECIFIED_SOURCE ( 'ANY', '', #7708, .NOT_KNOWN. ) ;
#9883=AXIS2_PLACEMENT_3D ( 'NONE', #10021, #17103, #9825 ) ;
#9922=ORIENTED_EDGE ( 'NONE', *, *, #14954, .T. ) ;
#9925=DIRECTION ( 'NONE',  ( -1.000000000000000000, 0.000000000000000000, 0.000000000000000000 ) ) ;
#9935=DIRECTION ( 'NONE',  ( 0.000000000000000000, 0.000000000000000000, 1.000000000000000000 ) ) ;
#9939=EDGE_CURVE ( 'NONE', #3542, #14183, #15713, .T. ) ;
#9945=CIRCLE ( 'NONE', #13634, 5.000000000000000888 ) ;
#10011=VECTOR ( 'NONE', #3371, 1000.000000000000000 ) ;
#10013=DIRECTION ( 'NONE',  ( 0.000000000000000000, 0.000000000000000000, -1.000000000000000000 ) ) ;
#10021=CARTESIAN_POINT ( 'NONE',  ( -199.9999999999999716, 9.999999999999973355, 6.000000000000000000 ) ) ;
#10072=EDGE_CURVE ( 'NONE', #400, #8123, #12943, .T. ) ;
#10086=VERTEX_POINT ( 'NONE', #1485 ) ;
#10132=DIRECTION ( 'NONE',  ( -1.000000000000000000, -0.000000000000000000, -0.000000000000000000 ) ) ;
#10165=DIRECTION ( 'NONE',  ( -1.000000000000000000, 0.000000000000000000, 0.000000000000000000 ) ) ;
#10175=CARTESIAN_POINT ( 'NONE',  ( -199.9999999999999716, 0.000000000000000000, -2.000000000000000000 ) ) ;
#10185=ORIENTED_EDGE ( 'NONE', *, *, #12688, .F. ) ;
#10226=AXIS2_PLACEMENT_3D ( 'NONE', #10384, #14677, #4179 ) ;
#10242=VECTOR ( 'NONE', #15838, 1000.000000000000000 ) ;
#10253=DIRECTION ( 'NONE',  ( 0.000000000000000000, 0.000000000000000000, 1.000000000000000000 ) ) ;
#10267=CARTESIAN_POINT ( 'NONE',  ( -66.35602477868049220, 4.999999999999973355, 11.00000000000000000 ) ) ;
#10269=EDGE_CURVE ( 'NONE', #5087, #18124, #4835, .T. ) ;
#10326=CARTESIAN_POINT ( 'NONE',  ( -194.9999999999999716, 4.999999999999973355, 6.000000000000005329 ) ) ;
#10364=SURFACE_SIDE_STYLE ('',( #10560 ) ) ;
#10384=CARTESIAN_POINT ( 'NONE',  ( -194.9999999999999716, 4.999999999999973355, 11.00000000000000000 ) ) ;
#10388=DIRECTION ( 'NONE',  ( 0.000000000000000000, 0.000000000000000000, 1.000000000000000000 ) ) ;
#10455=VERTEX_POINT ( 'NONE', #3809 ) ;
#10469=DIRECTION ( 'NONE',  ( 1.000000000000000000, 0.000000000000000000, 0.000000000000000000 ) ) ;
#10480=LINE ( 'NONE', #3198, #6876 ) ;
#10503=CARTESIAN_POINT ( 'NONE',  ( -205.0000000000000000, -5.000000000000024869, 3.000000000000002665 ) ) ;
#10560=SURFACE_STYLE_FILL_AREA ( #4729 ) ;
#10577=ORIENTED_EDGE ( 'NONE', *, *, #18476, .T. ) ;
#10657=LINE ( 'NONE', #12182, #10011 ) ;
#10662=DIRECTION ( 'NONE',  ( 0.000000000000000000, 1.000000000000000000, 0.000000000000000000 ) ) ;
#10673=ORIENTED_EDGE ( 'NONE', *, *, #4539, .T. ) ;
#10679=ORIENTED_EDGE ( 'NONE', *, *, #195, .F. ) ;
#10729=CIRCLE ( 'NONE', #17126, 5.000000000000004441 ) ;
#10766=CIRCLE ( 'NONE', #15620, 5.000000000000000000 ) ;
#10775=CARTESIAN_POINT ( 'NONE',  ( -205.0000000000000000, 4.999999999999975131, -153.7432847437423789 ) ) ;
#10802=DIRECTION ( 'NONE',  ( 1.000000000000000000, 0.000000000000000000, 0.000000000000000000 ) ) ;
#10807=DIRECTION ( 'NONE',  ( -1.000000000000000000, 0.000000000000000000, 0.000000000000000000 ) ) ;
#10818=EDGE_LOOP ( 'NONE', ( #17115, #18858, #7215, #778, #4865, #1393 ) ) ;
#10848=FACE_OUTER_BOUND ( 'NONE', #7221, .T. ) ;
#10867=VERTEX_POINT ( 'NONE', #6573 ) ;
#10875=VECTOR ( 'NONE', #15529, 1000.000000000000000 ) ;
#10950=VECTOR ( 'NONE', #3360, 1000.000000000000000 ) ;
#10971=EDGE_CURVE ( 'NONE', #18304, #10455, #18393, .T. ) ;
#11014=CYLINDRICAL_SURFACE ( 'NONE', #7179, 5.000000000000004441 ) ;
#11088=CARTESIAN_POINT ( 'NONE',  ( -194.9999999999999716, -5.000000000000024869, 3.000000000000002665 ) ) ;
#11149=ADVANCED_FACE ( 'NONE', ( #8929 ), #14757, .T. ) ;
#11155=CARTESIAN_POINT ( 'NONE',  ( -66.35602477868049220, -10.00000000000000888, 3.000000000000002665 ) ) ;
#11181=CIRCLE ( 'NONE', #4157, 5.000000000000004441 ) ;
#11192=ORIENTED_EDGE ( 'NONE', *, *, #17252, .F. ) ;
#11197=ORIENTED_EDGE ( 'NONE', *, *, #13631, .F. ) ;
#11223=ORIENTED_EDGE ( 'NONE', *, *, #4614, .F. ) ;
#11233=LINE ( 'NONE', #4047, #3488 ) ;
#11248=DIRECTION ( 'NONE',  ( 0.000000000000000000, 0.000000000000000000, 1.000000000000000000 ) ) ;
#11279=VERTEX_POINT ( 'NONE', #18382 ) ;
#11281=EDGE_CURVE ( 'NONE', #2507, #996, #4682, .T. ) ;
#11295=ADVANCED_FACE ( 'NONE', ( #12643 ), #2417, .T. ) ;
#11306=FACE_OUTER_BOUND ( 'NONE', #4982, .T. ) ;
#11355=ADVANCED_FACE ( 'NONE', ( #17133 ), #18653, .T. ) ;
#11365=VERTEX_POINT ( 'NONE', #15794 ) ;
#11395=VERTEX_POINT ( 'NONE', #1263 ) ;
#11396=CARTESIAN_POINT ( 'NONE',  ( -61.35602477868047799, 9.999999999999973355, 3.000000000000002665 ) ) ;
#11398=VECTOR ( 'NONE', #3070, 1000.000000000000000 ) ;
#11403=CIRCLE ( 'NONE', #107, 10.00000000000000888 ) ;
#11444=ORIENTED_EDGE ( 'NONE', *, *, #15609, .T. ) ;
#11453=ORIENTED_EDGE ( 'NONE', *, *, #7881, .T. ) ;
#11457=FACE_OUTER_BOUND ( 'NONE', #15136, .T. ) ;
#11511=ORIENTED_EDGE ( 'NONE', *, *, #13631, .T. ) ;
#11521=FACE_OUTER_BOUND ( 'NONE', #13883, .T. ) ;
#11524=CARTESIAN_POINT ( 'NONE',  ( -194.9999999999999716, -5.000000000000024869, 6.000000000000005329 ) ) ;
#11546=AXIS2_PLACEMENT_3D ( 'NONE', #18850, #5742, #18748 ) ;
#11562=AXIS2_PLACEMENT_3D ( 'NONE', #12839, #13030, #10165 ) ;
#11574=LINE ( 'NONE', #17392, #5580 ) ;
#11613=SHAPE_REPRESENTATION_RELATIONSHIP ( 'NONE' , 'NONE' ,  #16816, #17679 ) ;
#11629=ORIENTED_EDGE ( 'NONE', *, *, #11281, .F. ) ;
#11695=FACE_OUTER_BOUND ( 'NONE', #8234, .T. ) ;
#11704=DIRECTION ( 'NONE',  ( 0.000000000000000000, -1.000000000000000000, 0.000000000000000000 ) ) ;
#11714=CIRCLE ( 'NONE', #8363, 4.999999999999997335 ) ;
#11732=EDGE_CURVE ( 'NONE', #8583, #15844, #11574, .T. ) ;
#11740=ORIENTED_EDGE ( 'NONE', *, *, #4238, .T. ) ;
#11743=ORIENTED_EDGE ( 'NONE', *, *, #13287, .F. ) ;
#11752=CARTESIAN_POINT ( 'NONE',  ( -194.9999999999999716, 4.999999999999973355, 6.000000000000000000 ) ) ;
#11774=TOROIDAL_SURFACE ( 'NONE', #4443, 5.000000000000005329, 5.000000000000000000 ) ;
#11783=CYLINDRICAL_SURFACE ( 'NONE', #11546, 5.000000000000000000 ) ;
#11861=ORIENTED_EDGE ( 'NONE', *, *, #10072, .T. ) ;
#11879=ADVANCED_FACE ( 'NONE', ( #17589 ), #7441, .T. ) ;
#11938=EDGE_CURVE ( 'NONE', #8583, #14839, #921, .T. ) ;
#11944=VERTEX_POINT ( 'NONE', #5224 ) ;
#11967=EDGE_CURVE ( 'NONE', #10086, #2296, #741, .T. ) ;
#11968=EDGE_CURVE ( 'NONE', #14367, #400, #18707, .T. ) ;
#12074=EDGE_CURVE ( 'NONE', #14367, #10086, #11403, .T. ) ;
#12083=AXIS2_PLACEMENT_3D ( 'NONE', #18795, #8576, #13063 ) ;
#12112=DIRECTION ( 'NONE',  ( 1.000000000000000000, 1.239088197126290570E-16, -0.000000000000000000 ) ) ;
#12158=AXIS2_PLACEMENT_3D ( 'NONE', #7908, #13717, #632 ) ;
#12182=CARTESIAN_POINT ( 'NONE',  ( -205.0000000000000000, -5.000000000000024869, -153.7432847437423789 ) ) ;
#12183=ORIENTED_EDGE ( 'NONE', *, *, #5050, .T. ) ;
#12241=DIRECTION ( 'NONE',  ( 0.000000000000000000, 0.000000000000000000, -1.000000000000000000 ) ) ;
#12245=DIRECTION ( 'NONE',  ( -1.000000000000000000, -0.000000000000000000, -0.000000000000000000 ) ) ;
#12276=FACE_OUTER_BOUND ( 'NONE', #10818, .T. ) ;
#12333=ORIENTED_EDGE ( 'NONE', *, *, #12074, .T. ) ;
#12340=DIRECTION ( 'NONE',  ( 0.000000000000000000, 0.000000000000000000, -1.000000000000000000 ) ) ;
#12347=LINE ( 'NONE', #5177, #14540 ) ;
#12355=VECTOR ( 'NONE', #6565, 1000.000000000000000 ) ;
#12357=DIRECTION ( 'NONE',  ( -1.000000000000000000, 0.000000000000000000, -0.000000000000000000 ) ) ;
#12367=EDGE_CURVE ( 'NONE', #17792, #14367, #8723, .T. ) ;
#12419=VECTOR ( 'NONE', #5643, 1000.000000000000000 ) ;
#12484=DIRECTION ( 'NONE',  ( 1.000000000000000000, -0.000000000000000000, -0.000000000000000000 ) ) ;
#12488=EDGE_LOOP ( 'NONE', ( #6161, #7409, #5297, #11511, #11192, #9867 ) ) ;
#12524=CIRCLE ( 'NONE', #17365, 5.000000000000004441 ) ;
#12550=DIRECTION ( 'NONE',  ( -1.000000000000000000, -1.298018465182616140E-16, -0.000000000000000000 ) ) ;
#12581=FACE_OUTER_BOUND ( 'NONE', #18320, .T. ) ;
#12592=DIRECTION ( 'NONE',  ( 0.000000000000000000, 0.000000000000000000, -1.000000000000000000 ) ) ;
#12610=CARTESIAN_POINT ( 'NONE',  ( -194.9999999999999716, -5.000000000000024869, -153.7432847437423789 ) ) ;
#12643=FACE_OUTER_BOUND ( 'NONE', #7818, .T. ) ;
#12675=ORIENTED_EDGE ( 'NONE', *, *, #129, .F. ) ;
#12676=AXIS2_PLACEMENT_3D ( 'NONE', #6947, #4260, #5575 ) ;
#12688=EDGE_CURVE ( 'NONE', #4997, #18304, #14149, .T. ) ;
#12694=CIRCLE ( 'NONE', #4458, 5.000000000000004441 ) ;
#12702=DIRECTION ( 'NONE',  ( -1.000000000000000000, 0.000000000000000000, 0.000000000000000000 ) ) ;
#12747=EDGE_LOOP ( 'NONE', ( #10185, #11444, #1558, #11453 ) ) ;
#12753=ORIENTED_EDGE ( 'NONE', *, *, #9404, .F. ) ;
#12839=CARTESIAN_POINT ( 'NONE',  ( -194.9999999999999716, -5.000000000000024869, -2.000000000000000000 ) ) ;
#12842=VERTEX_POINT ( 'NONE', #16456 ) ;
#12849=DIRECTION ( 'NONE',  ( -0.000000000000000000, -0.000000000000000000, -1.000000000000000000 ) ) ;
#12921=VECTOR ( 'NONE', #14581, 1000.000000000000000 ) ;
#12934=CIRCLE ( 'NONE', #5307, 5.000000000000000000 ) ;
#12943=LINE ( 'NONE', #7416, #3829 ) ;
#12951=VERTEX_POINT ( 'NONE', #7637 ) ;
#12964=FACE_OUTER_BOUND ( 'NONE', #3214, .T. ) ;
#12993=ORIENTED_EDGE ( 'NONE', *, *, #14954, .F. ) ;
#13030=DIRECTION ( 'NONE',  ( 0.000000000000000000, 0.000000000000000000, -1.000000000000000000 ) ) ;
#13063=DIRECTION ( 'NONE',  ( 1.000000000000000000, -2.775557561562892929E-15, 0.000000000000000000 ) ) ;
#13080=CARTESIAN_POINT ( 'NONE',  ( -194.9999999999999716, 9.999999999999973355, 11.00000000000000000 ) ) ;
#13083=DIRECTION ( 'NONE',  ( -1.000000000000000000, 0.000000000000000000, 0.000000000000000000 ) ) ;
#13090=EDGE_CURVE ( 'NONE', #11279, #14839, #15069, .T. ) ;
#13095=ORIENTED_EDGE ( 'NONE', *, *, #3384, .F. ) ;
#13097=AXIS2_PLACEMENT_3D ( 'NONE', #12610, #9657, #6429 ) ;
#13116=CARTESIAN_POINT ( 'NONE',  ( -194.9999999999999716, 14.99999999999997513, 3.000000000000002665 ) ) ;
#13144=ORIENTED_EDGE ( 'NONE', *, *, #14077, .F. ) ;
#13174=FACE_OUTER_BOUND ( 'NONE', #15758, .T. ) ;
#13203=DIRECTION ( 'NONE',  ( 0.000000000000000000, -0.000000000000000000, 1.000000000000000000 ) ) ;
#13217=DIRECTION ( 'NONE',  ( 0.000000000000000000, 0.000000000000000000, -1.000000000000000000 ) ) ;
#13222=EDGE_CURVE ( 'NONE', #4747, #4298, #2460, .T. ) ;
#13241=EDGE_LOOP ( 'NONE', ( #4671, #3728, #8594, #12183 ) ) ;
#13247=CARTESIAN_POINT ( 'NONE',  ( -66.35602477868047799, 14.99999999999997513, 5.999999999999999112 ) ) ;
#13268=FACE_OUTER_BOUND ( 'NONE', #14411, .T. ) ;
#13275=EDGE_CURVE ( 'NONE', #996, #4997, #9196, .T. ) ;
#13287=EDGE_CURVE ( 'NONE', #15356, #5087, #763, .T. ) ;
#13300=DIRECTION ( 'NONE',  ( 0.000000000000000000, 1.000000000000000000, 0.000000000000000000 ) ) ;
#13327=FILL_AREA_STYLE_COLOUR ( '', #15149 ) ;
#13397=EDGE_CURVE ( 'NONE', #14839, #12951, #9811, .T. ) ;
#13412=CIRCLE ( 'NONE', #7635, 5.000000000000004441 ) ;
#13414=PLANE ( 'NONE',  #1290 ) ;
#13424=SURFACE_SIDE_STYLE ('',( #5865 ) ) ;
#13429=CARTESIAN_POINT ( 'NONE',  ( -66.35602477868049220, 14.99999999999997513, -153.7432847437423789 ) ) ;
#13436=CARTESIAN_POINT ( 'NONE',  ( -61.35602477868047799, 9.999999999999973355, -153.7432847437423789 ) ) ;
#13444=EDGE_CURVE ( 'NONE', #7533, #11395, #10729, .T. ) ;
#13473=CARTESIAN_POINT ( 'NONE',  ( -199.9999999999999716, 4.999999999999974243, 5.999999999999999112 ) ) ;
#13527=AXIS2_PLACEMENT_3D ( 'NONE', #7517, #3672, #3284 ) ;
#13544=LINE ( 'NONE', #5035, #16433 ) ;
#13549=ADVANCED_FACE ( 'NONE', ( #6102 ), #1799, .T. ) ;
#13585=CIRCLE ( 'NONE', #2580, 5.000000000000000000 ) ;
#13631=EDGE_CURVE ( 'NONE', #7533, #3542, #13544, .T. ) ;
#13634=AXIS2_PLACEMENT_3D ( 'NONE', #5482, #17149, #8458 ) ;
#13680=CARTESIAN_POINT ( 'NONE',  ( -194.9999999999999716, 9.999999999999973355, 6.000000000000000000 ) ) ;
#13717=DIRECTION ( 'NONE',  ( 1.000000000000000000, 0.000000000000000000, -0.000000000000000000 ) ) ;
#13758=CARTESIAN_POINT ( 'NONE',  ( -66.35602477868049220, -10.00000000000000888, 5.999999999999999112 ) ) ;
#13759=DIRECTION ( 'NONE',  ( -1.000000000000000000, 0.000000000000000000, 0.000000000000000000 ) ) ;
#13783=ORIENTED_EDGE ( 'NONE', *, *, #4670, .T. ) ;
#13797=CARTESIAN_POINT ( 'NONE',  ( -199.9999999999999716, 4.999999999999974243, 3.000000000000000000 ) ) ;
#13811=EDGE_CURVE ( 'NONE', #12951, #1583, #15532, .T. ) ;
#13817=LINE ( 'NONE', #733, #12355 ) ;
#13830=ORIENTED_EDGE ( 'NONE', *, *, #4688, .T. ) ;
#13845=CYLINDRICAL_SURFACE ( 'NONE', #16662, 5.000000000000000888 ) ;
#13847=DIRECTION ( 'NONE',  ( -0.000000000000000000, -0.000000000000000000, 1.000000000000000000 ) ) ;
#13864=FACE_OUTER_BOUND ( 'NONE', #13241, .T. ) ;
#13880=DIRECTION ( 'NONE',  ( 0.000000000000000000, 0.000000000000000000, -1.000000000000000000 ) ) ;
#13883=EDGE_LOOP ( 'NONE', ( #10577, #18590, #13095, #12993 ) ) ;
#13896=CIRCLE ( 'NONE', #18475, 4.999999999999997335 ) ;
#13905=ORIENTED_EDGE ( 'NONE', *, *, #8435, .F. ) ;
#13912=EDGE_CURVE ( 'NONE', #2507, #4747, #3084, .T. ) ;
#13921=AXIS2_PLACEMENT_3D ( 'NONE', #2365, #3798, #5235 ) ;
#13949=CARTESIAN_POINT ( 'NONE',  ( -194.9999999999999716, 4.999999999999973355, 3.000000000000002665 ) ) ;
#14077=EDGE_CURVE ( 'NONE', #10867, #18304, #1460, .T. ) ;
#14091=CIRCLE ( 'NONE', #681, 5.000000000000000000 ) ;
#14107=EDGE_LOOP ( 'NONE', ( #18103, #14206, #6355, #125 ) ) ;
#14130=VECTOR ( 'NONE', #3234, 1000.000000000000000 ) ;
#14149=LINE ( 'NONE', #1053, #15003 ) ;
#14181=ORIENTED_EDGE ( 'NONE', *, *, #4096, .F. ) ;
#14183=VERTEX_POINT ( 'NONE', #17134 ) ;
#14196=DIRECTION ( 'NONE',  ( -0.000000000000000000, 1.000000000000000000, 0.000000000000000000 ) ) ;
#14206=ORIENTED_EDGE ( 'NONE', *, *, #4614, .T. ) ;
#14216=VERTEX_POINT ( 'NONE', #13116 ) ;
#14268=ADVANCED_FACE ( 'NONE', ( #121 ), #11783, .T. ) ;
#14270=LINE ( 'NONE', #1169, #4749 ) ;
#14272=ORIENTED_EDGE ( 'NONE', *, *, #12367, .T. ) ;
#14280=ORIENTED_EDGE ( 'NONE', *, *, #5610, .F. ) ;
#14301=EDGE_CURVE ( 'NONE', #14216, #10086, #4812, .T. ) ;
#14318=DIRECTION ( 'NONE',  ( 0.000000000000000000, -0.000000000000000000, -1.000000000000000000 ) ) ;
#14329=DIRECTION ( 'NONE',  ( 0.000000000000000000, 1.000000000000000000, 0.000000000000000000 ) ) ;
#14342=ORIENTED_EDGE ( 'NONE', *, *, #14301, .T. ) ;
#14367=VERTEX_POINT ( 'NONE', #8223 ) ;
#14411=EDGE_LOOP ( 'NONE', ( #1702, #17709, #3655, #18122 ) ) ;
#14430=PRODUCT_DEFINITION ( 'UNKNOWN', '', #9874, #9242 ) ;
#14446=PLANE ( 'NONE',  #16013 ) ;
#14448=VECTOR ( 'NONE', #12484, 1000.000000000000000 ) ;
#14476=AXIS2_PLACEMENT_3D ( 'NONE', #15944, #8786, #2933 ) ;
#14519=DIRECTION ( 'NONE',  ( 0.000000000000000000, 0.000000000000000000, -1.000000000000000000 ) ) ;
#14531=VECTOR ( 'NONE', #10662, 1000.000000000000000 ) ;
#14540=VECTOR ( 'NONE', #2308, 1000.000000000000000 ) ;
#14581=DIRECTION ( 'NONE',  ( 0.000000000000000000, 0.000000000000000000, 1.000000000000000000 ) ) ;
#14593=CARTESIAN_POINT ( 'NONE',  ( -194.9999999999999716, 4.999999999999973355, 3.000000000000000000 ) ) ;
#14595=EDGE_LOOP ( 'NONE', ( #17896, #13905, #9496, #4700 ) ) ;
#14598=ADVANCED_FACE ( 'NONE', ( #4573 ), #4375, .T. ) ;
#14609=CIRCLE ( 'NONE', #11562, 5.000000000000004441 ) ;
#14639=FACE_OUTER_BOUND ( 'NONE', #3041, .T. ) ;
#14651=DIRECTION ( 'NONE',  ( -0.000000000000000000, -0.000000000000000000, 1.000000000000000000 ) ) ;
#14677=DIRECTION ( 'NONE',  ( 0.000000000000000000, 0.000000000000000000, 1.000000000000000000 ) ) ;
#14705=CARTESIAN_POINT ( 'NONE',  ( -194.9999999999999716, -5.000000000000024869, 11.00000000000000000 ) ) ;
#14713=AXIS2_PLACEMENT_3D ( 'NONE', #4432, #13217, #2318 ) ;
#14727=PLANE ( 'NONE',  #6582 ) ;
#14743=DIRECTION ( 'NONE',  ( -1.000000000000000000, 0.000000000000000000, 0.000000000000000000 ) ) ;
#14745=ORIENTED_EDGE ( 'NONE', *, *, #71, .T. ) ;
#14749=AXIS2_PLACEMENT_3D ( 'NONE', #13473, #14811, #6576 ) ;
#14757=PLANE ( 'NONE',  #13527 ) ;
#14810=CIRCLE ( 'NONE', #8117, 5.000000000000000000 ) ;
#14811=DIRECTION ( 'NONE',  ( 0.000000000000000000, 1.000000000000000000, -0.000000000000000000 ) ) ;
#14817=ORIENTED_EDGE ( 'NONE', *, *, #8212, .F. ) ;
#14839=VERTEX_POINT ( 'NONE', #5409 ) ;
#14904=CARTESIAN_POINT ( 'NONE',  ( -66.35602477868049220, -10.00000000000000888, 5.999999999999999112 ) ) ;
#14954=EDGE_CURVE ( 'NONE', #2296, #11365, #16306, .T. ) ;
#14959=DIRECTION ( 'NONE',  ( 0.000000000000000000, -1.000000000000000000, 0.000000000000000000 ) ) ;
#14980=DIRECTION ( 'NONE',  ( -0.000000000000000000, -1.000000000000000000, -0.000000000000000000 ) ) ;
#14982=DIRECTION ( 'NONE',  ( 1.000000000000000000, 0.000000000000000000, 2.775557561562892929E-15 ) ) ;
#14983=ORIENTED_EDGE ( 'NONE', *, *, #16559, .F. ) ;
#14986=VERTEX_POINT ( 'NONE', #7520 ) ;
#14989=AXIS2_PLACEMENT_3D ( 'NONE', #8039, #13847, #10807 ) ;
#15003=VECTOR ( 'NONE', #6895, 1000.000000000000000 ) ;
#15046=AXIS2_PLACEMENT_3D ( 'NONE', #3954, #5384, #16860 ) ;
#15064=CARTESIAN_POINT ( 'NONE',  ( -199.9999999999999716, -5.000000000000024869, 11.00000000000000000 ) ) ;
#15069=LINE ( 'NONE', #6567, #18346 ) ;
#15123=VECTOR ( 'NONE', #8686, 1000.000000000000000 ) ;
#15136=EDGE_LOOP ( 'NONE', ( #947, #11223, #1498, #18809 ) ) ;
#15141=ORIENTED_EDGE ( 'NONE', *, *, #16559, .T. ) ;
#15142=DIRECTION ( 'NONE',  ( 1.000000000000000000, 1.298018465182616140E-16, -0.000000000000000000 ) ) ;
#15149=COLOUR_RGB ( '', 0.08235294, 0.09019608, 0.10196078) ;
#15184=ORIENTED_EDGE ( 'NONE', *, *, #9213, .T. ) ;
#15192=DIRECTION ( 'NONE',  ( 0.000000000000000000, 0.000000000000000000, -1.000000000000000000 ) ) ;
#15199=VECTOR ( 'NONE', #14196, 1000.000000000000000 ) ;
#15247=LINE ( 'NONE', #6748, #3584 ) ;
#15286=DIRECTION ( 'NONE',  ( 1.000000000000000000, 0.000000000000000000, 0.000000000000000000 ) ) ;
#15289=ORIENTED_EDGE ( 'NONE', *, *, #949, .T. ) ;
#15325=CARTESIAN_POINT ( 'NONE',  ( -199.9999999999999716, -10.00000000000002665, 6.000000000000000000 ) ) ;
#15356=VERTEX_POINT ( 'NONE', #1465 ) ;
#15377=ORIENTED_EDGE ( 'NONE', *, *, #10971, .T. ) ;
#15382=AXIS2_PLACEMENT_3D ( 'NONE', #16126, #7436, #168 ) ;
#15436=DIRECTION ( 'NONE',  ( 0.000000000000000000, 0.000000000000000000, 1.000000000000000000 ) ) ;
#15465=DIRECTION ( 'NONE',  ( -0.000000000000000000, 1.000000000000000000, 0.000000000000000000 ) ) ;
#15468=CARTESIAN_POINT ( 'NONE',  ( -194.9999999999999716, 14.99999999999997513, -153.7432847437423789 ) ) ;
#15502=CARTESIAN_POINT ( 'NONE',  ( 0.000000000000000000, 0.000000000000000000, -2.000000000000000000 ) ) ;
#15529=DIRECTION ( 'NONE',  ( -0.000000000000000000, -0.000000000000000000, 1.000000000000000000 ) ) ;
#15532=LINE ( 'NONE', #5669, #15199 ) ;
#15534=CIRCLE ( 'NONE', #8075, 5.000000000000004441 ) ;
#15605=CARTESIAN_POINT ( 'NONE',  ( -194.9999999999999716, -15.00000000000003020, 3.000000000000002665 ) ) ;
#15609=EDGE_CURVE ( 'NONE', #4997, #4745, #18365, .T. ) ;
#15620=AXIS2_PLACEMENT_3D ( 'NONE', #7607, #16098, #6063 ) ;
#15624=ORIENTED_EDGE ( 'NONE', *, *, #5264, .T. ) ;
#15658=CARTESIAN_POINT ( 'NONE',  ( -66.35602477868049220, -15.00000000000001066, 3.000000000000002665 ) ) ;
#15660=ORIENTED_EDGE ( 'NONE', *, *, #13912, .T. ) ;
#15713=LINE ( 'NONE', #6945, #10875 ) ;
#15716=CARTESIAN_POINT ( 'NONE',  ( 0.000000000000000000, 0.000000000000000000, 0.000000000000000000 ) ) ;
#15758=EDGE_LOOP ( 'NONE', ( #17799, #7336, #14280, #7740 ) ) ;
#15794=CARTESIAN_POINT ( 'NONE',  ( -66.35602477868047799, 14.99999999999997513, 3.000000000000002665 ) ) ;
#15805=ORIENTED_EDGE ( 'NONE', *, *, #17252, .T. ) ;
#15838=DIRECTION ( 'NONE',  ( 1.000000000000000000, -0.000000000000000000, -0.000000000000000000 ) ) ;
#15844=VERTEX_POINT ( 'NONE', #13680 ) ;
#15944=CARTESIAN_POINT ( 'NONE',  ( -66.35602477868047799, -10.00000000000000888, 5.999999999999999112 ) ) ;
#15972=DIRECTION ( 'NONE',  ( -1.000000000000000000, 0.000000000000000000, -0.000000000000000000 ) ) ;
#15990=ORIENTED_EDGE ( 'NONE', *, *, #71, .F. ) ;
#16000=ADVANCED_FACE ( 'NONE', ( #8135 ), #8450, .T. ) ;
#16013=AXIS2_PLACEMENT_3D ( 'NONE', #1355, #7198, #15972 ) ;
#16033=VECTOR ( 'NONE', #12550, 1000.000000000000000 ) ;
#16034=CIRCLE ( 'NONE', #7823, 5.000000000000000000 ) ;
#16098=DIRECTION ( 'NONE',  ( -0.000000000000000000, 1.000000000000000000, -0.000000000000000000 ) ) ;
#16106=ADVANCED_FACE ( 'NONE', ( #11457 ), #1317, .T. ) ;
#16126=CARTESIAN_POINT ( 'NONE',  ( -66.35602477868047799, 9.999999999999973355, 5.999999999999999112 ) ) ;
#16152=DIRECTION ( 'NONE',  ( 0.000000000000000000, 0.000000000000000000, 1.000000000000000000 ) ) ;
#16163=CIRCLE ( 'NONE', #3953, 5.000000000000004441 ) ;
#16189=FACE_OUTER_BOUND ( 'NONE', #12488, .T. ) ;
#16236=ORIENTED_EDGE ( 'NONE', *, *, #11938, .F. ) ;
#16249=FACE_OUTER_BOUND ( 'NONE', #17328, .T. ) ;
#16263=CARTESIAN_POINT ( 'NONE',  ( -66.35602477868047799, -10.00000000000000888, 5.999999999999999112 ) ) ;
#16302=SURFACE_STYLE_USAGE ( .BOTH. , #13424 ) ;
#16306=LINE ( 'NONE', #13429, #2929 ) ;
#16343=FACE_OUTER_BOUND ( 'NONE', #5466, .T. ) ;
#16374=ORIENTED_EDGE ( 'NONE', *, *, #645, .F. ) ;
#16396=PRESENTATION_STYLE_ASSIGNMENT (( #3076 ) ) ;
#16404=( LENGTH_UNIT ( ) NAMED_UNIT ( * ) SI_UNIT ( .MILLI., .METRE. ) );
#16423=DIRECTION ( 'NONE',  ( 0.000000000000000000, -1.000000000000000000, 0.000000000000000000 ) ) ;
#16430=DIRECTION ( 'NONE',  ( 0.000000000000000000, 0.000000000000000000, -1.000000000000000000 ) ) ;
#16433=VECTOR ( 'NONE', #14980, 1000.000000000000000 ) ;
#16456=CARTESIAN_POINT ( 'NONE',  ( -66.35602477868049220, -15.00000000000001066, 5.999999999999999112 ) ) ;
#16550=CARTESIAN_POINT ( 'NONE',  ( -199.9999999999999716, 9.999999999999973355, 3.000000000000000000 ) ) ;
#16559=EDGE_CURVE ( 'NONE', #11365, #15356, #2349, .T. ) ;
#16662=AXIS2_PLACEMENT_3D ( 'NONE', #5334, #15465, #18066 ) ;
#16668=MANIFOLD_SOLID_BREP ( 'Cavity1', #4189 ) ;
#16816=SHAPE_REPRESENTATION ( 'Soft-Grip Handle Sleeve Overmolds (x2)', ( #2030 ), #5983 ) ;
#16846=ORIENTED_EDGE ( 'NONE', *, *, #4670, .F. ) ;
#16860=DIRECTION ( 'NONE',  ( 0.000000000000000000, 0.000000000000000000, 1.000000000000000000 ) ) ;
#16870=ORIENTED_EDGE ( 'NONE', *, *, #2425, .F. ) ;
#16888=ORIENTED_EDGE ( 'NONE', *, *, #13222, .T. ) ;
#16903=FACE_OUTER_BOUND ( 'NONE', #4725, .T. ) ;
#16952=SHAPE_DEFINITION_REPRESENTATION ( #368, #16816 ) ;
#17064=EDGE_CURVE ( 'NONE', #4298, #14216, #3326, .T. ) ;
#17066=ADVANCED_FACE ( 'NONE', ( #18176 ), #2213, .T. ) ;
#17103=DIRECTION ( 'NONE',  ( 0.000000000000000000, -1.000000000000000000, 0.000000000000000000 ) ) ;
#17115=ORIENTED_EDGE ( 'NONE', *, *, #13090, .F. ) ;
#17126=AXIS2_PLACEMENT_3D ( 'NONE', #14593, #1512, #17858 ) ;
#17133=FACE_OUTER_BOUND ( 'NONE', #729, .T. ) ;
#17134=CARTESIAN_POINT ( 'NONE',  ( -199.9999999999999716, -5.000000000000024869, 6.000000000000000000 ) ) ;
#17149=DIRECTION ( 'NONE',  ( -0.000000000000000000, 1.000000000000000000, 0.000000000000000000 ) ) ;
#17210=ORIENTED_EDGE ( 'NONE', *, *, #9146, .F. ) ;
#17217=AXIS2_PLACEMENT_3D ( 'NONE', #6305, #17873, #4585 ) ;
#17249=DIRECTION ( 'NONE',  ( 1.000000000000000000, 0.000000000000000000, 0.000000000000000000 ) ) ;
#17252=EDGE_CURVE ( 'NONE', #879, #3542, #12524, .T. ) ;
#17264=DIRECTION ( 'NONE',  ( 0.000000000000000000, 0.000000000000000000, -1.000000000000000000 ) ) ;
#17291=FACE_OUTER_BOUND ( 'NONE', #3005, .T. ) ;
#17297=AXIS2_PLACEMENT_3D ( 'NONE', #7695, #6901, #9672 ) ;
#17328=EDGE_LOOP ( 'NONE', ( #456, #2401, #14983 ) ) ;
#17340=CARTESIAN_POINT ( 'NONE',  ( -66.35602477868047799, 9.999999999999973355, -153.7432847437423789 ) ) ;
#17365=AXIS2_PLACEMENT_3D ( 'NONE', #18626, #14519, #4086 ) ;
#17383=FACE_OUTER_BOUND ( 'NONE', #17550, .T. ) ;
#17392=CARTESIAN_POINT ( 'NONE',  ( -199.9999999999999716, 9.999999999999973355, 6.000000000000000000 ) ) ;
#17396=EDGE_LOOP ( 'NONE', ( #6751, #16236, #6017, #17210 ) ) ;
#17424=ORIENTED_EDGE ( 'NONE', *, *, #13287, .T. ) ;
#17480=CARTESIAN_POINT ( 'NONE',  ( -194.9999999999999716, -10.00000000000002665, 3.000000000000002665 ) ) ;
#17523=CYLINDRICAL_SURFACE ( 'NONE', #14713, 5.000000000000004441 ) ;
#17525=EDGE_LOOP ( 'NONE', ( #2265, #12675, #18078, #6805 ) ) ;
#17535=AXIS2_PLACEMENT_3D ( 'NONE', #11752, #7270, #13083 ) ;
#17550=EDGE_LOOP ( 'NONE', ( #6003, #4897, #16846, #6975 ) ) ;
#17589=FACE_OUTER_BOUND ( 'NONE', #14595, .T. ) ;
#17632=FILL_AREA_STYLE_COLOUR ( '', #830 ) ;
#17679=ADVANCED_BREP_SHAPE_REPRESENTATION ( '', ( #16668, #2030 ), #5983 ) ;
#17709=ORIENTED_EDGE ( 'NONE', *, *, #10072, .F. ) ;
#17792=VERTEX_POINT ( 'NONE', #4062 ) ;
#17799=ORIENTED_EDGE ( 'NONE', *, *, #11732, .T. ) ;
#17836=AXIS2_PLACEMENT_3D ( 'NONE', #10775, #9925, #8685 ) ;
#17858=DIRECTION ( 'NONE',  ( -1.000000000000000000, 0.000000000000000000, 0.000000000000000000 ) ) ;
#17861=DIRECTION ( 'NONE',  ( 0.000000000000000000, 1.000000000000000000, -0.000000000000000000 ) ) ;
#17873=DIRECTION ( 'NONE',  ( 0.000000000000000000, -1.000000000000000000, 0.000000000000000000 ) ) ;
#17893=DIRECTION ( 'NONE',  ( 0.000000000000000000, -0.000000000000000000, -1.000000000000000000 ) ) ;
#17896=ORIENTED_EDGE ( 'NONE', *, *, #11968, .T. ) ;
#17945=ORIENTED_EDGE ( 'NONE', *, *, #9939, .T. ) ;
#18011=EDGE_LOOP ( 'NONE', ( #10679, #6357, #4763, #15377 ) ) ;
#18066=DIRECTION ( 'NONE',  ( 0.000000000000000000, 0.000000000000000000, 1.000000000000000000 ) ) ;
#18078=ORIENTED_EDGE ( 'NONE', *, *, #13090, .T. ) ;
#18086=DIRECTION ( 'NONE',  ( -1.000000000000000000, 0.000000000000000000, 0.000000000000000000 ) ) ;
#18103=ORIENTED_EDGE ( 'NONE', *, *, #12367, .F. ) ;
#18122=ORIENTED_EDGE ( 'NONE', *, *, #5943, .F. ) ;
#18124=VERTEX_POINT ( 'NONE', #1436 ) ;
#18176=FACE_OUTER_BOUND ( 'NONE', #18011, .T. ) ;
#18192=PLANE ( 'NONE',  #9419 ) ;
#18217=ADVANCED_FACE ( 'NONE', ( #17291 ), #2752, .T. ) ;
#18253=CARTESIAN_POINT ( 'NONE',  ( -66.35602477868047799, 0.000000000000000000, -2.000000000000000000 ) ) ;
#18292=LINE ( 'NONE', #15325, #12419 ) ;
#18304=VERTEX_POINT ( 'NONE', #4686 ) ;
#18320=EDGE_LOOP ( 'NONE', ( #7430, #4553, #2359, #746, #8718, #11861 ) ) ;
#18328=ORIENTED_EDGE ( 'NONE', *, *, #18440, .F. ) ;
#18346=VECTOR ( 'NONE', #7828, 1000.000000000000000 ) ;
#18365=LINE ( 'NONE', #5179, #4501 ) ;
#18382=CARTESIAN_POINT ( 'NONE',  ( -194.9999999999999716, -10.00000000000002665, 6.000000000000000000 ) ) ;
#18387=DIRECTION ( 'NONE',  ( -0.000000000000000000, 1.000000000000000000, -0.000000000000000000 ) ) ;
#18393=CIRCLE ( 'NONE', #7427, 10.00000000000000888 ) ;
#18406=ADVANCED_FACE ( 'NONE', ( #16903 ), #13845, .T. ) ;
#18410=PLANE ( 'NONE',  #10226 ) ;
#18440=EDGE_CURVE ( 'NONE', #204, #12842, #14810, .T. ) ;
#18465=ADVANCED_FACE ( 'NONE', ( #4970 ), #11774, .T. ) ;
#18475=AXIS2_PLACEMENT_3D ( 'NONE', #3808, #8037, #15286 ) ;
#18476=EDGE_CURVE ( 'NONE', #2296, #8583, #13896, .T. ) ;
#18488=DIRECTION ( 'NONE',  ( 0.000000000000000000, 0.000000000000000000, 1.000000000000000000 ) ) ;
#18557=EDGE_LOOP ( 'NONE', ( #3219, #8185, #13144, #14181 ) ) ;
#18589=EDGE_CURVE ( 'NONE', #4298, #15356, #2641, .T. ) ;
#18590=ORIENTED_EDGE ( 'NONE', *, *, #1312, .F. ) ;
#18591=ADVANCED_FACE ( 'NONE', ( #12964 ), #5791, .T. ) ;
#18606=CARTESIAN_POINT ( 'NONE',  ( 0.000000000000000000, 9.999999999999973355, -2.000000000000000000 ) ) ;
#18611=CARTESIAN_POINT ( 'NONE',  ( -199.9999999999999716, -5.000000000000024869, 6.000000000000005329 ) ) ;
#18620=CARTESIAN_POINT ( 'NONE',  ( -199.9999999999999716, 4.999999999999973355, 3.000000000000000000 ) ) ;
#18626=CARTESIAN_POINT ( 'NONE',  ( -194.9999999999999716, -5.000000000000024869, 3.000000000000000000 ) ) ;
#18648=DIRECTION ( 'NONE',  ( 1.000000000000000000, 1.298018465182616140E-16, -0.000000000000000000 ) ) ;
#18653=CYLINDRICAL_SURFACE ( 'NONE', #5285, 10.00000000000000888 ) ;
#18664=LINE ( 'NONE', #1563, #11398 ) ;
#18683=ORIENTED_EDGE ( 'NONE', *, *, #9051, .F. ) ;
#18707=CIRCLE ( 'NONE', #14749, 5.000000000000000000 ) ;
#18710=DIRECTION ( 'NONE',  ( 0.000000000000000000, 0.000000000000000000, 1.000000000000000000 ) ) ;
#18748=DIRECTION ( 'NONE',  ( 0.000000000000000000, 0.000000000000000000, 1.000000000000000000 ) ) ;
#18758=AXIS2_PLACEMENT_3D ( 'NONE', #4114, #8511, #9935 ) ;
#18795=CARTESIAN_POINT ( 'NONE',  ( -66.35602477868047799, -10.00000000000000888, 3.000000000000000000 ) ) ;
#18809=ORIENTED_EDGE ( 'NONE', *, *, #13912, .F. ) ;
#18850=CARTESIAN_POINT ( 'NONE',  ( -66.35602477868049220, 4.999999999999973355, 5.999999999999999112 ) ) ;
#18858=ORIENTED_EDGE ( 'NONE', *, *, #723, .F. ) ;
#18898=ADVANCED_FACE ( 'NONE', ( #7126 ), #5358, .T. ) ;
ENDSEC;
END-ISO-10303-21;
